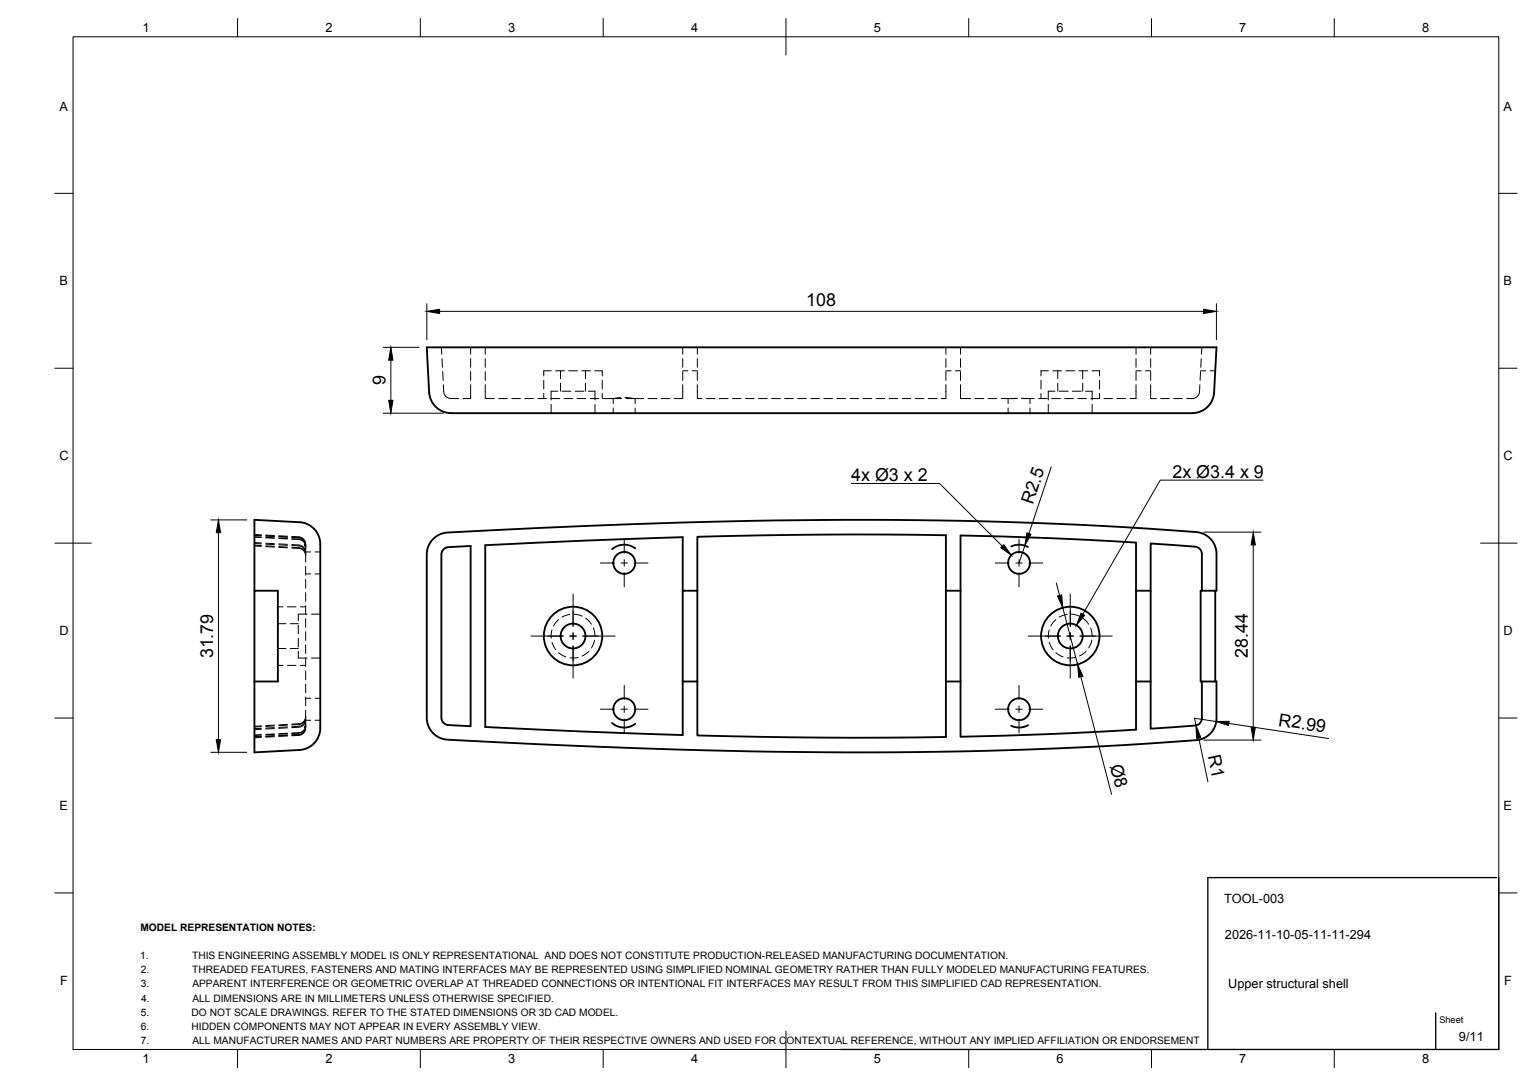
ISO-10303-21;
HEADER;
/* Generated by software containing ST-Developer
 * from STEP Tools, Inc. (www.steptools.com) 
 */

FILE_DESCRIPTION(
/* description */ (''),
/* implementation_level */ '2;1');

FILE_NAME(
/* name */ 'Upper structural shell.step',
/* time_stamp */ '2026-11-10T05:20:16-08:00',
/* author */ (''),
/* organization */ (''),
/* preprocessor_version */ 'ST-DEVELOPER v20.2',
/* originating_system */ 'Autodesk Translation Framework v15.17.0.0',
/* authorisation */ '');

FILE_SCHEMA (('AUTOMOTIVE_DESIGN { 1 0 10303 214 3 1 1 }'));
ENDSEC;

DATA;
#10=MECHANICAL_DESIGN_GEOMETRIC_PRESENTATION_REPRESENTATION('',(#116),#24809);
#76=SPHERICAL_SURFACE('',#10334,0.1);
#77=SPHERICAL_SURFACE('',#10337,0.0999999999999998);
#78=SPHERICAL_SURFACE('',#10341,0.0999999999999993);
#79=SPHERICAL_SURFACE('',#10345,0.1);
#80=SPHERICAL_SURFACE('',#10350,0.3);
#81=SPHERICAL_SURFACE('',#10354,0.3);
#82=SPHERICAL_SURFACE('',#10358,0.299999999999999);
#83=SPHERICAL_SURFACE('',#10363,0.3);
#96=SHAPE_REPRESENTATION_RELATIONSHIP('SRR','None',#24860,#106);
#106=ADVANCED_BREP_SHAPE_REPRESENTATION('',(#126),#24803);
#116=STYLED_ITEM('',(#24922),#126);
#126=MANIFOLD_SOLID_BREP('Body1',#9893);
#147=FACE_BOUND('',#2104,.T.);
#148=FACE_BOUND('',#2105,.T.);
#149=FACE_BOUND('',#2106,.T.);
#150=FACE_BOUND('',#2113,.T.);
#151=FACE_BOUND('',#2116,.T.);
#152=FACE_BOUND('',#2127,.T.);
#153=FACE_BOUND('',#2129,.T.);
#154=FACE_BOUND('',#2141,.T.);
#155=FACE_BOUND('',#2162,.T.);
#156=FACE_BOUND('',#2163,.T.);
#157=FACE_BOUND('',#2164,.T.);
#158=FACE_BOUND('',#2199,.T.);
#159=FACE_BOUND('',#2200,.T.);
#160=FACE_BOUND('',#2201,.T.);
#161=FACE_BOUND('',#2202,.T.);
#162=FACE_BOUND('',#2203,.T.);
#163=FACE_BOUND('',#2204,.T.);
#205=B_SPLINE_SURFACE_WITH_KNOTS('',3,3,((#15043,#15044,#15045,#15046),
(#15047,#15048,#15049,#15050),(#15051,#15052,#15053,#15054),(#15055,#15056,
#15057,#15058),(#15059,#15060,#15061,#15062)),.UNSPECIFIED.,.F.,.F.,.F.,
(4,1,4),(4,4),(0.,0.571428571428571,1.),(1.0454440030657,3.44967454744645),
 .UNSPECIFIED.);
#206=B_SPLINE_SURFACE_WITH_KNOTS('',3,3,((#15135,#15136,#15137,#15138),
(#15139,#15140,#15141,#15142),(#15143,#15144,#15145,#15146),(#15147,#15148,
#15149,#15150),(#15151,#15152,#15153,#15154)),.UNSPECIFIED.,.F.,.F.,.F.,
(4,1,4),(4,4),(0.,0.571428571428571,1.),(7.24519303641511,9.95046872158573),
 .UNSPECIFIED.);
#207=B_SPLINE_SURFACE_WITH_KNOTS('',3,3,((#16016,#16017,#16018,#16019),
(#16020,#16021,#16022,#16023),(#16024,#16025,#16026,#16027),(#16028,#16029,
#16030,#16031)),.UNSPECIFIED.,.F.,.F.,.F.,(4,4),(4,4),(0.0705535719740953,
0.323522444336189),(0.0117434863834119,0.684857763552191),.UNSPECIFIED.);
#208=B_SPLINE_SURFACE_WITH_KNOTS('',3,3,((#16036,#16037,#16038,#16039),
(#16040,#16041,#16042,#16043),(#16044,#16045,#16046,#16047),(#16048,#16049,
#16050,#16051)),.UNSPECIFIED.,.F.,.F.,.F.,(4,4),(4,4),(0.0262419052680539,
0.0545428296147404),(0.0121538053864343,0.684980602226481),
 .UNSPECIFIED.);
#209=B_SPLINE_SURFACE_WITH_KNOTS('',3,3,((#16061,#16062,#16063,#16064),
(#16065,#16066,#16067,#16068),(#16069,#16070,#16071,#16072),(#16073,#16074,
#16075,#16076),(#16077,#16078,#16079,#16080)),.UNSPECIFIED.,.F.,.F.,.F.,
(4,1,4),(4,4),(0.,0.571428571428571,1.),(0.752061768057538,3.45733745322815),
 .UNSPECIFIED.);
#210=B_SPLINE_SURFACE_WITH_KNOTS('',3,3,((#16081,#16082,#16083,#16084),
(#16085,#16086,#16087,#16088),(#16089,#16090,#16091,#16092),(#16093,#16094,
#16095,#16096),(#16097,#16098,#16099,#16100)),.UNSPECIFIED.,.F.,.F.,.F.,
(4,1,4),(4,4),(0.,0.571428571428571,1.),(0.283259008618247,0.557056952888827),
 .UNSPECIFIED.);
#211=B_SPLINE_SURFACE_WITH_KNOTS('',3,3,((#16114,#16115,#16116,#16117),
(#16118,#16119,#16120,#16121),(#16122,#16123,#16124,#16125),(#16126,#16127,
#16128,#16129)),.UNSPECIFIED.,.F.,.F.,.F.,(4,4),(4,4),(0.67647755566375,
0.929446428026011),(0.0117434863436937,0.684857763580381),.UNSPECIFIED.);
#212=B_SPLINE_SURFACE_WITH_KNOTS('',3,3,((#16130,#16131,#16132,#16133),
(#16134,#16135,#16136,#16137),(#16138,#16139,#16140,#16141),(#16142,#16143,
#16144,#16145)),.UNSPECIFIED.,.F.,.F.,.F.,(4,4),(4,4),(0.945457170385156,
0.973758094731946),(0.0121538053598088,0.684980602226481),.UNSPECIFIED.);
#213=B_SPLINE_SURFACE_WITH_KNOTS('',3,3,((#16229,#16230,#16231,#16232),
(#16233,#16234,#16235,#16236),(#16237,#16238,#16239,#16240),(#16241,#16242,
#16243,#16244)),.UNSPECIFIED.,.F.,.F.,.F.,(4,4),(4,4),(0.341142793678372,
0.658675488550287),(0.0116221239297273,0.684255166525269),.UNSPECIFIED.);
#214=B_SPLINE_SURFACE_WITH_KNOTS('',3,3,((#16249,#16250,#16251,#16252),
(#16253,#16254,#16255,#16256),(#16257,#16258,#16259,#16260),(#16261,#16262,
#16263,#16264),(#16265,#16266,#16267,#16268)),.UNSPECIFIED.,.F.,.F.,.F.,
(4,1,4),(4,4),(0.,0.571428571428571,1.),(3.65450559744172,7.0548588409572),
 .UNSPECIFIED.);
#215=B_SPLINE_SURFACE_WITH_KNOTS('',3,3,((#16278,#16279,#16280,#16281),
(#16282,#16283,#16284,#16285),(#16286,#16287,#16288,#16289),(#16290,#16291,
#16292,#16293),(#16294,#16295,#16296,#16297)),.UNSPECIFIED.,.F.,.F.,.F.,
(4,1,4),(4,4),(0.,0.571428571428571,1.),(3.64767164868607,7.04802489220155),
 .UNSPECIFIED.);
#216=B_SPLINE_SURFACE_WITH_KNOTS('',3,3,((#16302,#16303,#16304,#16305),
(#16306,#16307,#16308,#16309),(#16310,#16311,#16312,#16313),(#16314,#16315,
#16316,#16317)),.UNSPECIFIED.,.F.,.F.,.F.,(4,4),(4,4),(0.341324511449716,
0.658857206321627),(0.0116221214776208,0.684255166525269),.UNSPECIFIED.);
#217=B_SPLINE_SURFACE_WITH_KNOTS('',3,3,((#16362,#16363,#16364,#16365),
(#16366,#16367,#16368,#16369),(#16370,#16371,#16372,#16373),(#16374,#16375,
#16376,#16377)),.UNSPECIFIED.,.F.,.F.,.F.,(4,4),(4,4),(0.676316266718331,
0.901708040522105),(0.0117102006467275,0.68495201331719),.UNSPECIFIED.);
#218=B_SPLINE_SURFACE_WITH_KNOTS('',3,3,((#16382,#16383,#16384,#16385),
(#16386,#16387,#16388,#16389),(#16390,#16391,#16392,#16393),(#16394,#16395,
#16396,#16397),(#16398,#16399,#16400,#16401)),.UNSPECIFIED.,.F.,.F.,.F.,
(4,1,4),(4,4),(0.,0.571428571428571,1.),(7.25285594219682,9.65708648657758),
 .UNSPECIFIED.);
#219=B_SPLINE_SURFACE_WITH_KNOTS('',3,3,((#16411,#16412,#16413,#16414),
(#16415,#16416,#16417,#16418),(#16419,#16420,#16421,#16422),(#16423,#16424,
#16425,#16426)),.UNSPECIFIED.,.F.,.F.,.F.,(4,4),(4,4),(0.0982919594778951,
0.323683733281714),(0.0117102006467272,0.68495201331719),.UNSPECIFIED.);
#220=B_SPLINE_SURFACE_WITH_KNOTS('',3,3,((#16501,#16502,#16503,#16504),
(#16505,#16506,#16507,#16508),(#16509,#16510,#16511,#16512),(#16513,#16514,
#16515,#16516)),.UNSPECIFIED.,.F.,.F.,.F.,(4,4),(4,4),(0.917922863855343,
0.974411608827007),(0.0122403473423911,0.685344304754238),.UNSPECIFIED.);
#221=B_SPLINE_SURFACE_WITH_KNOTS('',3,3,((#16526,#16527,#16528,#16529),
(#16530,#16531,#16532,#16533),(#16534,#16535,#16536,#16537),(#16538,#16539,
#16540,#16541),(#16542,#16543,#16544,#16545)),.UNSPECIFIED.,.F.,.F.,.F.,
(4,1,4),(4,4),(0.,0.571428571428571,1.),(9.85085636625011,10.4271318523291),
 .UNSPECIFIED.);
#222=B_SPLINE_SURFACE_WITH_KNOTS('',3,3,((#16559,#16560,#16561,#16562),
(#16563,#16564,#16565,#16566),(#16567,#16568,#16569,#16570),(#16571,#16572,
#16573,#16574)),.UNSPECIFIED.,.F.,.F.,.F.,(4,4),(4,4),(0.025588391172993,
0.0820771361446569),(0.0122403473423911,0.685344304754238),
 .UNSPECIFIED.);
#223=B_SPLINE_SURFACE_WITH_KNOTS('',3,3,((#16584,#16585,#16586,#16587),
(#16588,#16589,#16590,#16591),(#16592,#16593,#16594,#16595),(#16596,#16597,
#16598,#16599),(#16600,#16601,#16602,#16603)),.UNSPECIFIED.,.F.,.F.,.F.,
(4,1,4),(4,4),(0.,0.571428571428571,1.),(0.27539863731415,0.851674123393175),
 .UNSPECIFIED.);
#224=B_SPLINE_SURFACE_WITH_KNOTS('',3,3,((#16617,#16618,#16619,#16620),
(#16621,#16622,#16623,#16624),(#16625,#16626,#16627,#16628),(#16629,#16630,
#16631,#16632),(#16633,#16634,#16635,#16636)),.UNSPECIFIED.,.F.,.F.,.F.,
(4,1,4),(4,4),(0.,0.571428571428571,1.),(0.00944995813270487,0.618489359031386),
 .UNSPECIFIED.);
#225=B_SPLINE_SURFACE_WITH_KNOTS('',3,3,((#16643,#16644,#16645,#16646),
(#16647,#16648,#16649,#16650),(#16651,#16652,#16653,#16654),(#16655,#16656,
#16657,#16658),(#16659,#16660,#16661,#16662)),.UNSPECIFIED.,.F.,.F.,.F.,
(4,1,4),(4,4),(0.,0.571428571428571,1.),(0.00908570715245136,0.618164468641375),
 .UNSPECIFIED.);
#226=B_SPLINE_SURFACE_WITH_KNOTS('',3,3,((#16667,#16668,#16669,#16670),
(#16671,#16672,#16673,#16674),(#16675,#16676,#16677,#16678),(#16679,#16680,
#16681,#16682),(#16683,#16684,#16685,#16686)),.UNSPECIFIED.,.F.,.F.,.F.,
(4,1,4),(4,4),(0.,0.571428571428571,1.),(0.0091183540525243,0.618164468641375),
 .UNSPECIFIED.);
#227=B_SPLINE_SURFACE_WITH_KNOTS('',3,3,((#16691,#16692,#16693,#16694),
(#16695,#16696,#16697,#16698),(#16699,#16700,#16701,#16702),(#16703,#16704,
#16705,#16706),(#16707,#16708,#16709,#16710)),.UNSPECIFIED.,.F.,.F.,.F.,
(4,1,4),(4,4),(0.,0.571428571428571,1.),(10.1454735367545,10.419271481025),
 .UNSPECIFIED.);
#228=B_SPLINE_SURFACE_WITH_KNOTS('',3,3,((#16711,#16712,#16713,#16714),
(#16715,#16716,#16717,#16718),(#16719,#16720,#16721,#16722),(#16723,#16724,
#16725,#16726),(#16727,#16728,#16729,#16730)),.UNSPECIFIED.,.F.,.F.,.F.,
(4,1,4),(4,4),(0.,0.571428571428571,1.),(0.0094045468285345,0.618489359031386),
 .UNSPECIFIED.);
#229=B_SPLINE_SURFACE_WITH_KNOTS('',3,3,((#16756,#16757,#16758,#16759),
(#16760,#16761,#16762,#16763),(#16764,#16765,#16766,#16767),(#16768,#16769,
#16770,#16771),(#16772,#16773,#16774,#16775)),.UNSPECIFIED.,.F.,.F.,.F.,
(4,1,4),(4,4),(0.,0.571428571428571,1.),(-0.00535061636073277,0.618489359031386),
 .UNSPECIFIED.);
#230=B_SPLINE_SURFACE_WITH_KNOTS('',3,3,((#16794,#16795,#16796,#16797,#16798),
(#16799,#16800,#16801,#16802,#16803),(#16804,#16805,#16806,#16807,#16808),
(#16809,#16810,#16811,#16812,#16813),(#16814,#16815,#16816,#16817,#16818)),
 .UNSPECIFIED.,.F.,.F.,.F.,(4,1,4),(4,1,4),(0.,0.571428571428571,1.),(0.283259008618247,
4.63063308449434,10.4271318523291),.UNSPECIFIED.);
#231=B_SPLINE_SURFACE_WITH_KNOTS('',3,3,((#16829,#16830,#16831,#16832),
(#16833,#16834,#16835,#16836),(#16837,#16838,#16839,#16840),(#16841,#16842,
#16843,#16844),(#16845,#16846,#16847,#16848)),.UNSPECIFIED.,.F.,.F.,.F.,
(4,1,4),(4,4),(0.,0.571428571428571,1.),(-0.00578978989683084,0.618164468641375),
 .UNSPECIFIED.);
#232=B_SPLINE_SURFACE_WITH_KNOTS('',3,3,((#16857,#16858,#16859,#16860),
(#16861,#16862,#16863,#16864),(#16865,#16866,#16867,#16868),(#16869,#16870,
#16871,#16872),(#16873,#16874,#16875,#16876)),.UNSPECIFIED.,.F.,.F.,.F.,
(4,1,4),(4,4),(0.,0.571428571428571,1.),(-0.00569189159989896,0.618164468641375),
 .UNSPECIFIED.);
#233=B_SPLINE_SURFACE_WITH_KNOTS('',3,3,((#16885,#16886,#16887,#16888,#16889),
(#16890,#16891,#16892,#16893,#16894),(#16895,#16896,#16897,#16898,#16899),
(#16900,#16901,#16902,#16903,#16904),(#16905,#16906,#16907,#16908,#16909)),
 .UNSPECIFIED.,.F.,.F.,.F.,(4,1,4),(4,1,4),(0.,0.571428571428571,1.),(0.27539863731415,
4.62277271319024,10.419271481025),.UNSPECIFIED.);
#234=B_SPLINE_SURFACE_WITH_KNOTS('',3,3,((#16920,#16921,#16922,#16923),
(#16924,#16925,#16926,#16927),(#16928,#16929,#16930,#16931),(#16932,#16933,
#16934,#16935),(#16936,#16937,#16938,#16939)),.UNSPECIFIED.,.F.,.F.,.F.,
(4,1,4),(4,4),(0.,0.571428571428571,1.),(-0.0054868135546625,0.618489359031386),
 .UNSPECIFIED.);
#235=B_SPLINE_SURFACE_WITH_KNOTS('',3,3,((#16948,#16949,#16950,#16951),
(#16952,#16953,#16954,#16955),(#16956,#16957,#16958,#16959),(#16960,#16961,
#16962,#16963)),.UNSPECIFIED.,.F.,.F.,.F.,(4,4),(4,4),(0.026239262514127,
0.974414173651419),(0.,0.685344304754238),.UNSPECIFIED.);
#236=B_SPLINE_SURFACE_WITH_KNOTS('',3,3,((#16966,#16967,#16968,#16969),
(#16970,#16971,#16972,#16973),(#16974,#16975,#16976,#16977),(#16978,#16979,
#16980,#16981)),.UNSPECIFIED.,.F.,.F.,.F.,(4,4),(4,4),(0.0255858263485814,
0.973760737485873),(0.,0.685344304754238),.UNSPECIFIED.);
#617=B_SPLINE_CURVE_WITH_KNOTS('',3,(#14942,#14943,#14944,#14945,#14946,
#14947,#14948,#14949,#14950,#14951,#14952,#14953,#14954,#14955,#14956,#14957,
#14958,#14959,#14960,#14961,#14962,#14963,#14964,#14965),.UNSPECIFIED.,
 .F.,.F.,(4,2,2,2,2,2,2,2,2,2,2,4),(-0.337265338267783,-0.250544943628509,
-0.208272806508042,-0.186542211788094,-0.176382978682897,-0.170925844043069,
-0.16639450677335,-0.161077381235501,-0.15182241135393,-0.115009181549223,
-0.030206004227969,0.),.UNSPECIFIED.);
#618=B_SPLINE_CURVE_WITH_KNOTS('',3,(#14970,#14971,#14972,#14973,#14974,
#14975,#14976,#14977,#14978,#14979,#14980,#14981,#14982,#14983,#14984,#14985,
#14986,#14987,#14988,#14989),.UNSPECIFIED.,.F.,.F.,(4,2,2,2,2,2,2,2,2,4),
(-0.240982594686416,-0.16829976149504,-0.141836598208813,-0.129116059226128,
-0.121962912034391,-0.115857591426886,-0.108506552485159,-0.0948769875819265,
-0.0364654790774683,0.),.UNSPECIFIED.);
#619=B_SPLINE_CURVE_WITH_KNOTS('',3,(#14994,#14995,#14996,#14997,#14998,
#14999,#15000,#15001,#15002,#15003,#15004,#15005,#15006,#15007,#15008,#15009,
#15010,#15011,#15012,#15013),.UNSPECIFIED.,.F.,.F.,(4,2,2,2,2,2,2,2,2,4),
(-0.240981214998207,-0.168303541671295,-0.141841407502325,-0.129121097580905,
-0.121968013294536,-0.115862708924237,-0.108511643765797,-0.0948818976588229,
-0.0364681276985956,0.),.UNSPECIFIED.);
#620=B_SPLINE_CURVE_WITH_KNOTS('',3,(#15018,#15019,#15020,#15021,#15022,
#15023,#15024,#15025,#15026,#15027,#15028,#15029,#15030,#15031,#15032,#15033,
#15034,#15035,#15036,#15037,#15038,#15039,#15040,#15041),.UNSPECIFIED.,
 .F.,.F.,(4,2,2,2,2,2,2,2,2,2,2,4),(-0.337269388373684,-0.250545316912909,
-0.208282401844766,-0.186554569827561,-0.176396213396297,-0.17093921790305,
-0.16640782243471,-0.161090427650893,-0.151834477986603,-0.115010808423941,
-0.0302102096065556,0.),.UNSPECIFIED.);
#621=B_SPLINE_CURVE_WITH_KNOTS('',3,(#15064,#15065,#15066,#15067),
 .UNSPECIFIED.,.F.,.F.,(4,4),(1.0454440030657,2.52465537163019),
 .UNSPECIFIED.);
#622=B_SPLINE_CURVE_WITH_KNOTS('',3,(#15069,#15070,#15071,#15072,#15073,
#15074,#15075,#15076,#15077,#15078,#15079,#15080,#15081,#15082,#15083,#15084,
#15085,#15086,#15087,#15088,#15089,#15090,#15091,#15092,#15093,#15094,#15095,
#15096),.UNSPECIFIED.,.F.,.F.,(4,3,3,3,3,3,3,3,3,4),(-0.152193408756968,
-0.128427023368412,-0.115107736263918,-0.0911810900745799,-0.0780377802127556,
-0.0652031397886901,-0.0414031558437525,-0.0389949527774582,-0.0152076153333754,
0.),.UNSPECIFIED.);
#623=B_SPLINE_CURVE_WITH_KNOTS('',3,(#15098,#15099,#15100,#15101),
 .UNSPECIFIED.,.F.,.F.,(4,4),(-3.44967454744645,-1.05170160817356),
 .UNSPECIFIED.);
#624=B_SPLINE_CURVE_WITH_KNOTS('',3,(#15103,#15104,#15105,#15106,#15107,
#15108,#15109,#15110,#15111,#15112,#15113,#15114,#15115,#15116,#15117,#15118,
#15119,#15120,#15121,#15122,#15123,#15124,#15125,#15126,#15127,#15128,#15129,
#15130),.UNSPECIFIED.,.F.,.F.,(4,3,3,3,3,3,3,3,3,4),(-0.152278960443096,
-0.128503570101575,-0.115218572146868,-0.09145408274965,-0.0870214650669139,
-0.0781562978024333,-0.0542566895399357,-0.03908030849237,-0.0153296112319379,
0.),.UNSPECIFIED.);
#625=B_SPLINE_CURVE_WITH_KNOTS('',3,(#15131,#15132,#15133,#15134),
 .UNSPECIFIED.,.F.,.F.,(4,4),(2.75501813708031,3.4476340663212),
 .UNSPECIFIED.);
#626=B_SPLINE_CURVE_WITH_KNOTS('',3,(#15156,#15157,#15158,#15159),
 .UNSPECIFIED.,.F.,.F.,(4,4),(7.24810383506675,7.89761558728778),
 .UNSPECIFIED.);
#627=B_SPLINE_CURVE_WITH_KNOTS('',3,(#15161,#15162,#15163,#15164,#15165,
#15166,#15167,#15168,#15169,#15170,#15171,#15172,#15173,#15174,#15175,#15176,
#15177,#15178,#15179,#15180,#15181,#15182,#15183,#15184,#15185,#15186,#15187,
#15188),.UNSPECIFIED.,.F.,.F.,(4,3,3,3,3,3,3,3,3,4),(-0.152278869104567,
-0.128548794904564,-0.115192257893812,-0.0912773536606376,-0.0781090575823055,
-0.0652724057916263,-0.0414819581560496,-0.0390493575290778,-0.015259721743698,
0.),.UNSPECIFIED.);
#628=B_SPLINE_CURVE_WITH_KNOTS('',3,(#15190,#15191,#15192,#15193),
 .UNSPECIFIED.,.F.,.F.,(4,4),(-9.94532343034734,-7.24519303641511),
 .UNSPECIFIED.);
#629=B_SPLINE_CURVE_WITH_KNOTS('',3,(#15195,#15196,#15197,#15198,#15199,
#15200,#15201,#15202,#15203,#15204,#15205,#15206,#15207,#15208,#15209,#15210,
#15211,#15212,#15213,#15214,#15215,#15216,#15217,#15218,#15219,#15220,#15221,
#15222),.UNSPECIFIED.,.F.,.F.,(4,3,3,3,3,3,3,3,3,4),(-0.152181623618259,
-0.128410404494075,-0.115248188224843,-0.0914746846046984,-0.0869904866333268,
-0.0783028696190655,-0.0543945376065823,-0.0391651209697638,-0.0153884182770307,
0.),.UNSPECIFIED.);
#630=B_SPLINE_CURVE_WITH_KNOTS('',3,(#15223,#15224,#15225,#15226),
 .UNSPECIFIED.,.F.,.F.,(4,4),(8.21380824320284,9.95046871680089),
 .UNSPECIFIED.);
#631=B_SPLINE_CURVE_WITH_KNOTS('',3,(#15229,#15230,#15231,#15232),
 .UNSPECIFIED.,.F.,.F.,(4,4),(2.80491490332713,3.45442665446657),
 .UNSPECIFIED.);
#632=B_SPLINE_CURVE_WITH_KNOTS('',3,(#15236,#15237,#15238,#15239),
 .UNSPECIFIED.,.F.,.F.,(4,4),(0.752061768057538,2.48872224644044),
 .UNSPECIFIED.);
#633=B_SPLINE_CURVE_WITH_KNOTS('',3,(#15387,#15388,#15389,#15390,#15391,
#15392),.UNSPECIFIED.,.F.,.F.,(4,2,4),(-0.606700505977711,-0.303383635264422,
-0.000339350725729326),.UNSPECIFIED.);
#634=B_SPLINE_CURVE_WITH_KNOTS('',3,(#15393,#15394,#15395,#15396,#15397,
#15398,#15399,#15400,#15401,#15402,#15403,#15404,#15405,#15406,#15407,#15408,
#15409,#15410,#15411,#15412,#15413,#15414,#15415,#15416,#15417,#15418,#15419,
#15420),.UNSPECIFIED.,.F.,.F.,(4,3,3,3,3,3,3,3,3,4),(-0.152173579228948,
-0.128423230539522,-0.115115104157663,-0.0911927259648815,-0.0780672068328041,
-0.0652082609452843,-0.0414117413801899,-0.0390174000215468,-0.0152300060615686,
0.),.UNSPECIFIED.);
#635=B_SPLINE_CURVE_WITH_KNOTS('',3,(#15421,#15422,#15423,#15424,#15425,
#15426),.UNSPECIFIED.,.F.,.F.,(4,2,4),(-0.606471894652381,-0.303383500305553,
-0.00011071898471493),.UNSPECIFIED.);
#636=B_SPLINE_CURVE_WITH_KNOTS('',3,(#15430,#15431,#15432,#15433,#15434,
#15435),.UNSPECIFIED.,.F.,.F.,(4,2,4),(-0.606240625011114,-0.303433113375332,
-0.00010938105916114),.UNSPECIFIED.);
#637=B_SPLINE_CURVE_WITH_KNOTS('',3,(#15437,#15438,#15439,#15440,#15441,
#15442,#15443,#15444,#15445,#15446,#15447,#15448,#15449,#15450,#15451,#15452,
#15453,#15454,#15455,#15456,#15457,#15458,#15459,#15460,#15461,#15462,#15463,
#15464),.UNSPECIFIED.,.F.,.F.,(4,3,3,3,3,3,3,3,3,4),(-0.152281454644235,
-0.128508102092242,-0.115234945630277,-0.0914677943501604,-0.0870276017853555,
-0.0781846052914712,-0.0542821334115454,-0.0390966859411886,-0.0153419673568312,
0.),.UNSPECIFIED.);
#638=B_SPLINE_CURVE_WITH_KNOTS('',3,(#15466,#15467,#15468,#15469,#15470,
#15471),.UNSPECIFIED.,.F.,.F.,(4,2,4),(-0.606758573154242,-0.303433157101101,
-0.000627306481538803),.UNSPECIFIED.);
#639=B_SPLINE_CURVE_WITH_KNOTS('',3,(#15477,#15478,#15479,#15480,#15481,
#15482),.UNSPECIFIED.,.F.,.F.,(4,2,4),(-0.60617382748,-0.303436117212405,
-7.2700296824213E-5),.UNSPECIFIED.);
#640=B_SPLINE_CURVE_WITH_KNOTS('',3,(#15484,#15485,#15486,#15487,#15488,
#15489,#15490,#15491,#15492,#15493,#15494,#15495,#15496,#15497,#15498,#15499,
#15500,#15501,#15502,#15503,#15504,#15505,#15506,#15507,#15508,#15509,#15510,
#15511),.UNSPECIFIED.,.F.,.F.,(4,3,3,3,3,3,3,3,3,4),(-0.152282154327755,
-0.128558036203745,-0.115201429639692,-0.0912891813973639,-0.0781219052297615,
-0.065279687589213,-0.0414913146723999,-0.0390591331507366,-0.0152683745546824,
0.),.UNSPECIFIED.);
#641=B_SPLINE_CURVE_WITH_KNOTS('',3,(#15515,#15516,#15517,#15518,#15519,
#15520,#15521,#15522,#15523,#15524,#15525,#15526,#15527,#15528,#15529,#15530,
#15531,#15532,#15533,#15534,#15535,#15536,#15537,#15538,#15539,#15540,#15541,
#15542),.UNSPECIFIED.,.F.,.F.,(4,3,3,3,3,3,3,3,3,4),(-0.152283066055976,
-0.128508717930245,-0.115216472798554,-0.091451700383826,-0.087022506454752,
-0.0781485278686168,-0.0542483994686567,-0.0390758108455304,-0.0153274175274101,
0.),.UNSPECIFIED.);
#642=B_SPLINE_CURVE_WITH_KNOTS('',3,(#15544,#15545,#15546,#15547,#15548,
#15549),.UNSPECIFIED.,.F.,.F.,(4,2,4),(-0.606800264911061,-0.303436147592132,
-0.000699137727853738),.UNSPECIFIED.);
#643=B_SPLINE_CURVE_WITH_KNOTS('',3,(#15554,#15555,#15556,#15557,#15558,
#15559),.UNSPECIFIED.,.F.,.F.,(4,2,4),(-0.606915279655722,-0.30363236403835,
-0.000516487074480598),.UNSPECIFIED.);
#644=B_SPLINE_CURVE_WITH_KNOTS('',3,(#15563,#15564,#15565,#15566,#15567,
#15568,#15569,#15570,#15571,#15572,#15573,#15574,#15575,#15576,#15577,#15578,
#15579,#15580,#15581,#15582,#15583,#15584,#15585,#15586,#15587,#15588,#15589,
#15590),.UNSPECIFIED.,.F.,.F.,(4,3,3,3,3,3,3,3,3,4),(-0.152205325335401,
-0.128433618138404,-0.115304790388008,-0.091527299141506,-0.0870178586418932,
-0.0783866443643876,-0.0544751548276533,-0.0392137310602028,-0.0154203878854647,
0.),.UNSPECIFIED.);
#645=B_SPLINE_CURVE_WITH_KNOTS('',3,(#15592,#15593,#15594,#15595,#15596,
#15597),.UNSPECIFIED.,.F.,.F.,(4,2,4),(-0.606752424187958,-0.303632696349781,
-0.000353591088346872),.UNSPECIFIED.);
#646=B_SPLINE_CURVE_WITH_KNOTS('',3,(#15603,#15604,#15605,#15606),
 .UNSPECIFIED.,.F.,.F.,(4,4),(0.0116023361771303,0.618489359031386),
 .UNSPECIFIED.);
#647=B_SPLINE_CURVE_WITH_KNOTS('',3,(#15610,#15611,#15612,#15613),
 .UNSPECIFIED.,.F.,.F.,(4,4),(-0.618489359031386,-0.01160233617713),
 .UNSPECIFIED.);
#648=B_SPLINE_CURVE_WITH_KNOTS('',3,(#15616,#15617,#15618,#15619),
 .UNSPECIFIED.,.F.,.F.,(4,4),(7.01593971618694,9.71770560667459),
 .UNSPECIFIED.);
#649=B_SPLINE_CURVE_WITH_KNOTS('',3,(#15620,#15621,#15622,#15623),
 .UNSPECIFIED.,.F.,.F.,(4,4),(0.505945342046796,3.20718651982575),
 .UNSPECIFIED.);
#650=B_SPLINE_CURVE_WITH_KNOTS('',3,(#15626,#15627,#15628,#15629,#15630,
#15631,#15632),.UNSPECIFIED.,.F.,.F.,(4,3,4),(3.40717417387402,5.11170895874517,
6.80746068626633),.UNSPECIFIED.);
#651=B_SPLINE_CURVE_WITH_KNOTS('',3,(#15635,#15636,#15637,#15638),
 .UNSPECIFIED.,.F.,.F.,(4,4),(7.00766573366377,9.41198845520559),
 .UNSPECIFIED.);
#652=B_SPLINE_CURVE_WITH_KNOTS('',3,(#15642,#15643,#15644,#15645),
 .UNSPECIFIED.,.F.,.F.,(4,4),(9.61248784142317,10.2217363065808),
 .UNSPECIFIED.);
#653=B_SPLINE_CURVE_WITH_KNOTS('',3,(#15646,#15647,#15648,#15649,#15650,
#15651,#15652,#15653,#15654,#15655,#15656,#15657,#15658,#15659,#15660,#15661,
#15662,#15663,#15664,#15665,#15666,#15667,#15668,#15669,#15670,#15671,#15672,
#15673),.UNSPECIFIED.,.F.,.F.,(4,3,3,3,3,3,3,3,3,4),(0.,0.0238103109064959,
0.0390781362249314,0.0628635086275546,0.0641230352384255,0.0780643700703951,
0.101962174814111,0.113803522271848,0.137549611554782,0.149564734365165),
 .UNSPECIFIED.);
#654=B_SPLINE_CURVE_WITH_KNOTS('',3,(#15677,#15678,#15679,#15680,#15681,
#15682,#15683,#15684,#15685,#15686,#15687,#15688,#15689,#15690,#15691,#15692,
#15693,#15694,#15695,#15696,#15697,#15698,#15699,#15700,#15701,#15702,#15703,
#15704,#15705,#15706,#15707),.UNSPECIFIED.,.F.,.F.,(4,3,3,3,3,3,3,3,3,3,
4),(0.,0.0535521515156599,0.107729685495911,0.117233338918226,0.171447998942947,
0.1923696899792,0.234191611538245,0.288659693466396,0.341410301570312,0.395549383747909,
0.448696573746633),.UNSPECIFIED.);
#655=B_SPLINE_CURVE_WITH_KNOTS('',3,(#15709,#15710,#15711,#15712),
 .UNSPECIFIED.,.F.,.F.,(4,4),(0.0255858263485814,0.973760737485873),
 .UNSPECIFIED.);
#656=B_SPLINE_CURVE_WITH_KNOTS('',3,(#15714,#15715,#15716,#15717,#15718,
#15719,#15720,#15721,#15722,#15723,#15724,#15725,#15726,#15727,#15728,#15729,
#15730,#15731,#15732,#15733,#15734,#15735,#15736,#15737,#15738,#15739,#15740,
#15741,#15742,#15743,#15744),.UNSPECIFIED.,.F.,.F.,(4,3,3,3,3,3,3,3,3,3,
4),(0.,0.0535144560117858,0.107726856902975,0.117300577410231,0.171517675930231,
0.195438847090422,0.234297456941738,0.289665153342662,0.345032849743585,
0.40043206955427,0.455831289364955),.UNSPECIFIED.);
#657=B_SPLINE_CURVE_WITH_KNOTS('',3,(#15748,#15749,#15750,#15751,#15752,
#15753,#15754,#15755,#15756,#15757,#15758,#15759,#15760,#15761,#15762,#15763,
#15764,#15765,#15766,#15767,#15768,#15769,#15770,#15771,#15772,#15773,#15774,
#15775,#15776,#15777,#15778),.UNSPECIFIED.,.F.,.F.,(4,3,3,3,3,3,3,3,3,3,
4),(0.,0.053505543180391,0.107714168832353,0.117253997025819,0.171473395203321,
0.195418854185489,0.234223199196375,0.289607016015183,0.344990832833991,
0.400409777473312,0.455828722112633),.UNSPECIFIED.);
#658=B_SPLINE_CURVE_WITH_KNOTS('',3,(#15780,#15781,#15782,#15783),
 .UNSPECIFIED.,.F.,.F.,(4,4),(0.0262392625141271,0.974414173651419),
 .UNSPECIFIED.);
#659=B_SPLINE_CURVE_WITH_KNOTS('',3,(#15785,#15786,#15787,#15788,#15789,
#15790,#15791,#15792,#15793,#15794,#15795,#15796,#15797,#15798,#15799,#15800,
#15801,#15802,#15803,#15804,#15805,#15806,#15807,#15808,#15809,#15810,#15811,
#15812,#15813,#15814,#15815),.UNSPECIFIED.,.F.,.F.,(4,3,3,3,3,3,3,3,3,3,
4),(0.,0.0535648734523888,0.107747221190676,0.117299947751206,0.171510987106922,
0.192397607227928,0.234296687348373,0.288768001369001,0.341469499352622,
0.395597672314973,0.448700135162036),.UNSPECIFIED.);
#660=B_SPLINE_CURVE_WITH_KNOTS('',3,(#15818,#15819,#15820,#15821,#15822,
#15823,#15824,#15825,#15826,#15827,#15828,#15829,#15830,#15831,#15832,#15833,
#15834,#15835,#15836,#15837,#15838,#15839,#15840,#15841,#15842),
 .UNSPECIFIED.,.F.,.F.,(4,3,3,3,3,3,3,3,4),(0.,0.0238141989470671,0.0391004231578824,
0.0641320992313133,0.0780996136084711,0.101998806889826,0.113823260594808,
0.137564745199532,0.149565921982294),.UNSPECIFIED.);
#661=B_SPLINE_CURVE_WITH_KNOTS('',3,(#15844,#15845,#15846,#15847),
 .UNSPECIFIED.,.F.,.F.,(4,4),(2.76692059912875E-5,0.609394470571143),
 .UNSPECIFIED.);
#662=B_SPLINE_CURVE_WITH_KNOTS('',3,(#15850,#15851,#15852,#15853),
 .UNSPECIFIED.,.F.,.F.,(4,4),(0.809932799154201,3.21472245120952),
 .UNSPECIFIED.);
#663=B_SPLINE_CURVE_WITH_KNOTS('',3,(#15856,#15857,#15858,#15859,#15860,
#15861,#15862),.UNSPECIFIED.,.F.,.F.,(4,3,4),(3.41496637450242,5.11093193409745,
6.81591321610411),.UNSPECIFIED.);
#664=B_SPLINE_CURVE_WITH_KNOTS('',3,(#15866,#15867,#15868,#15869),
 .UNSPECIFIED.,.F.,.F.,(4,4),(9.91798263530139,10.2237206759544),
 .UNSPECIFIED.);
#665=B_SPLINE_CURVE_WITH_KNOTS('',3,(#15871,#15872,#15873,#15874,#15875,
#15876,#15877,#15878,#15879,#15880,#15881,#15882,#15883,#15884,#15885,#15886,
#15887,#15888,#15889,#15890,#15891,#15892,#15893,#15894,#15895,#15896,#15897,
#15898),.UNSPECIFIED.,.F.,.F.,(4,3,3,3,3,3,3,3,3,4),(0.,0.023807020713713,
0.039085080816122,0.0628703378723092,0.0651394887354207,0.0780750047750988,
0.101981498769656,0.114997221725907,0.138748569029605,0.151942344104828),
 .UNSPECIFIED.);
#666=B_SPLINE_CURVE_WITH_KNOTS('',3,(#15902,#15903,#15904,#15905,#15906,
#15907,#15908,#15909,#15910,#15911,#15912,#15913,#15914,#15915,#15916,#15917,
#15918,#15919,#15920,#15921,#15922,#15923,#15924,#15925,#15926,#15927,#15928,
#15929),.UNSPECIFIED.,.F.,.F.,(4,3,3,3,3,3,3,3,3,4),(0.,0.0238098191818892,
0.0391006681981376,0.0628849269680955,0.0651459659463291,0.0780999162396042,
0.102007524384594,0.115011225379555,0.138759376430353,0.151943200125079),
 .UNSPECIFIED.);
#667=B_SPLINE_CURVE_WITH_KNOTS('',3,(#15931,#15932,#15933,#15934),
 .UNSPECIFIED.,.F.,.F.,(4,4),(2.85486020485948E-5,0.305707210239178),
 .UNSPECIFIED.);
#668=B_SPLINE_CURVE_WITH_KNOTS('',3,(#15944,#15945,#15946,#15947,#15948,
#15949),.UNSPECIFIED.,.F.,.F.,(4,2,4),(-0.606446248197249,-0.303383959626182,
-6.4365448350312E-5),.UNSPECIFIED.);
#669=B_SPLINE_CURVE_WITH_KNOTS('',3,(#15951,#15952,#15953,#15954,#15955,
#15956),.UNSPECIFIED.,.F.,.F.,(4,2,4),(-0.60675170080159,-0.303384112192838,
-0.000369837888147484),.UNSPECIFIED.);
#670=B_SPLINE_CURVE_WITH_KNOTS('',3,(#15958,#15959,#15960,#15961,#15962,
#15963,#15964,#15965,#15966,#15967,#15968,#15969,#15970,#15971,#15972,#15973,
#15974,#15975,#15976,#15977,#15978,#15979,#15980,#15981,#15982,#15983,#15984,
#15985),.UNSPECIFIED.,.F.,.F.,(4,3,3,3,3,3,3,3,3,4),(-0.152162866344201,
-0.128411131698784,-0.115108013904405,-0.0911850729173883,-0.0780642464630149,
-0.0652023242402653,-0.0414053499882389,-0.0390151293250392,-0.0152279490549848,
0.),.UNSPECIFIED.);
#671=B_SPLINE_CURVE_WITH_KNOTS('',3,(#15988,#15989,#15990,#15991,#15992,
#15993,#15994,#15995,#15996,#15997,#15998,#15999,#16000,#16001,#16002,#16003,
#16004,#16005,#16006,#16007,#16008,#16009,#16010,#16011,#16012,#16013,#16014,
#16015),.UNSPECIFIED.,.F.,.F.,(4,3,3,3,3,3,3,3,3,4),(-0.152171297476962,
-0.128400300768352,-0.115247520946962,-0.0914735511738372,-0.0869860114952295,
-0.0783112904282795,-0.0544025203706761,-0.0391699941254272,-0.015391764586027,
0.),.UNSPECIFIED.);
#672=B_SPLINE_CURVE_WITH_KNOTS('',3,(#16032,#16033,#16034,#16035),
 .UNSPECIFIED.,.F.,.F.,(4,4),(-3.45733745322815,-0.757207059295936),
 .UNSPECIFIED.);
#673=B_SPLINE_CURVE_WITH_KNOTS('',3,(#16053,#16054,#16055,#16056),
 .UNSPECIFIED.,.F.,.F.,(4,4),(-0.557056952888827,-0.283259008618247),
 .UNSPECIFIED.);
#674=B_SPLINE_CURVE_WITH_KNOTS('',3,(#16057,#16058,#16059,#16060),
 .UNSPECIFIED.,.F.,.F.,(4,4),(-0.618164468641375,-0.0110156167597059),
 .UNSPECIFIED.);
#675=B_SPLINE_CURVE_WITH_KNOTS('',3,(#16102,#16103,#16104,#16105),
 .UNSPECIFIED.,.F.,.F.,(4,4),(0.283259011433088,0.551788488929761),
 .UNSPECIFIED.);
#676=B_SPLINE_CURVE_WITH_KNOTS('',3,(#16109,#16110,#16111,#16112),
 .UNSPECIFIED.,.F.,.F.,(4,4),(10.1507419987596,10.419271481025),
 .UNSPECIFIED.);
#677=B_SPLINE_CURVE_WITH_KNOTS('',3,(#16147,#16148,#16149,#16150),
 .UNSPECIFIED.,.F.,.F.,(4,4),(0.0110156167597055,0.618164468641375),
 .UNSPECIFIED.);
#678=B_SPLINE_CURVE_WITH_KNOTS('',3,(#16151,#16152,#16153,#16154),
 .UNSPECIFIED.,.F.,.F.,(4,4),(-10.419271481025,-10.1454735367545),
 .UNSPECIFIED.);
#679=B_SPLINE_CURVE_WITH_KNOTS('',3,(#16157,#16158,#16159,#16160,#16161,
#16162),.UNSPECIFIED.,.F.,.F.,(4,2,4),(-0.606211482799139,-0.303431960476852,
-9.19895310989571E-5),.UNSPECIFIED.);
#680=B_SPLINE_CURVE_WITH_KNOTS('',3,(#16164,#16165,#16166,#16167,#16168,
#16169,#16170,#16171,#16172,#16173,#16174,#16175,#16176,#16177,#16178,#16179,
#16180,#16181,#16182,#16183,#16184,#16185,#16186,#16187,#16188,#16189,#16190,
#16191),.UNSPECIFIED.,.F.,.F.,(4,3,3,3,3,3,3,3,3,4),(-0.152283340966725,
-0.128554242174982,-0.115196092098682,-0.0912819860997417,-0.0781117853096875,
-0.0652755629514801,-0.0414857317972147,-0.039051434275634,-0.0152612146291672,
0.),.UNSPECIFIED.);
#681=B_SPLINE_CURVE_WITH_KNOTS('',3,(#16195,#16196,#16197,#16198,#16199,
#16200,#16201,#16202,#16203,#16204,#16205,#16206,#16207,#16208,#16209,#16210,
#16211,#16212,#16213,#16214,#16215,#16216,#16217,#16218,#16219,#16220,#16221,
#16222),.UNSPECIFIED.,.F.,.F.,(4,3,3,3,3,3,3,3,3,4),(-0.152285570909379,
-0.128511627155755,-0.115232904621082,-0.0914664612111958,-0.0870286654075453,
-0.0781769338106538,-0.0542752301960614,-0.039092246575741,-0.0153386136911565,
0.),.UNSPECIFIED.);
#682=B_SPLINE_CURVE_WITH_KNOTS('',3,(#16223,#16224,#16225,#16226,#16227,
#16228),.UNSPECIFIED.,.F.,.F.,(4,2,4),(-0.606773318344362,-0.303431998667662,
-0.000653802131222458),.UNSPECIFIED.);
#683=B_SPLINE_CURVE_WITH_KNOTS('',3,(#16245,#16246,#16247,#16248),
 .UNSPECIFIED.,.F.,.F.,(4,4),(-7.05313168653828,-3.6572084986735),
 .UNSPECIFIED.);
#684=B_SPLINE_CURVE_WITH_KNOTS('',3,(#16269,#16270,#16271,#16272),
 .UNSPECIFIED.,.F.,.F.,(4,4),(3.65450559744172,7.0548588409572),
 .UNSPECIFIED.);
#685=B_SPLINE_CURVE_WITH_KNOTS('',3,(#16274,#16275,#16276,#16277),
 .UNSPECIFIED.,.F.,.F.,(4,4),(3.64767164868607,7.04802489220155),
 .UNSPECIFIED.);
#686=B_SPLINE_CURVE_WITH_KNOTS('',3,(#16298,#16299,#16300,#16301),
 .UNSPECIFIED.,.F.,.F.,(4,4),(-7.04532199096977,-3.64939880310499),
 .UNSPECIFIED.);
#687=B_SPLINE_CURVE_WITH_KNOTS('',3,(#16320,#16321,#16322,#16323,#16324,
#16325),.UNSPECIFIED.,.F.,.F.,(4,2,4),(-0.606200453641641,-0.30343602424441,
-9.0120313562092E-5),.UNSPECIFIED.);
#688=B_SPLINE_CURVE_WITH_KNOTS('',3,(#16327,#16328,#16329,#16330,#16331,
#16332,#16333,#16334,#16335,#16336,#16337,#16338,#16339,#16340,#16341,#16342,
#16343,#16344,#16345,#16346,#16347,#16348,#16349,#16350,#16351,#16352,#16353,
#16354),.UNSPECIFIED.,.F.,.F.,(4,3,3,3,3,3,3,3,3,4),(-0.152277688086818,
-0.128551334178815,-0.115197577176818,-0.0912856014461669,-0.0781191417238373,
-0.0652765169533013,-0.0414883027365163,-0.0390570310290822,-0.0152653090895913,
0.),.UNSPECIFIED.);
#689=B_SPLINE_CURVE_WITH_KNOTS('',3,(#16356,#16357,#16358,#16359,#16360,
#16361),.UNSPECIFIED.,.F.,.F.,(4,2,4),(-0.60678286609787,-0.303436074842897,
-0.000672492961417026),.UNSPECIFIED.);
#690=B_SPLINE_CURVE_WITH_KNOTS('',3,(#16378,#16379,#16380,#16381),
 .UNSPECIFIED.,.F.,.F.,(4,4),(-9.65082888146972,-7.25285594219682),
 .UNSPECIFIED.);
#691=B_SPLINE_CURVE_WITH_KNOTS('',3,(#16402,#16403,#16404,#16405),
 .UNSPECIFIED.,.F.,.F.,(4,4),(7.25489642332205,7.94751235889625),
 .UNSPECIFIED.);
#692=B_SPLINE_CURVE_WITH_KNOTS('',3,(#16406,#16407,#16408,#16409),
 .UNSPECIFIED.,.F.,.F.,(4,4),(8.17787511801303,9.65708648657758),
 .UNSPECIFIED.);
#693=B_SPLINE_CURVE_WITH_KNOTS('',3,(#16429,#16430,#16431,#16432,#16433,
#16434),.UNSPECIFIED.,.F.,.F.,(4,2,4),(-0.607007797795788,-0.303636495504298,
-0.000571323176327465),.UNSPECIFIED.);
#694=B_SPLINE_CURVE_WITH_KNOTS('',3,(#16436,#16437,#16438,#16439,#16440,
#16441,#16442,#16443,#16444,#16445,#16446,#16447,#16448,#16449,#16450,#16451,
#16452,#16453,#16454,#16455,#16456,#16457,#16458,#16459,#16460,#16461,#16462,
#16463),.UNSPECIFIED.,.F.,.F.,(4,3,3,3,3,3,3,3,3,4),(-0.152184339020145,
-0.128410461444444,-0.115096394428865,-0.0911692948751363,-0.0780261759644403,
-0.0651939085034322,-0.0413932235702045,-0.0389860720679279,-0.0151971168406065,
0.),.UNSPECIFIED.);
#695=B_SPLINE_CURVE_WITH_KNOTS('',3,(#16467,#16468,#16469,#16470,#16471,
#16472,#16473,#16474,#16475,#16476,#16477,#16478,#16479,#16480,#16481,#16482,
#16483,#16484,#16485,#16486,#16487,#16488,#16489,#16490,#16491,#16492,#16493,
#16494),.UNSPECIFIED.,.F.,.F.,(4,3,3,3,3,3,3,3,3,4),(-0.15219777746951,
-0.128424216118147,-0.115318679085322,-0.0915406112613293,-0.0870190514838729,
-0.0784197287877601,-0.0545085386658457,-0.0392329067084975,-0.0154317870320417,
0.),.UNSPECIFIED.);
#696=B_SPLINE_CURVE_WITH_KNOTS('',3,(#16495,#16496,#16497,#16498,#16499,
#16500),.UNSPECIFIED.,.F.,.F.,(4,2,4),(-0.606706256981509,-0.303636876939173,
-0.00026974181288697),.UNSPECIFIED.);
#697=B_SPLINE_CURVE_WITH_KNOTS('',3,(#16518,#16519,#16520,#16521),
 .UNSPECIFIED.,.F.,.F.,(4,4),(0.0112334529114386,0.618489359031386),
 .UNSPECIFIED.);
#698=B_SPLINE_CURVE_WITH_KNOTS('',3,(#16522,#16523,#16524,#16525),
 .UNSPECIFIED.,.F.,.F.,(4,4),(-10.4271318523291,-9.85085636625011),
 .UNSPECIFIED.);
#699=B_SPLINE_CURVE_WITH_KNOTS('',3,(#16548,#16549,#16550,#16551),
 .UNSPECIFIED.,.F.,.F.,(4,4),(9.85750350611301,10.4271318523291),
 .UNSPECIFIED.);
#700=B_SPLINE_CURVE_WITH_KNOTS('',3,(#16555,#16556,#16557,#16558),
 .UNSPECIFIED.,.F.,.F.,(4,4),(0.27539863731415,0.845026983530265),
 .UNSPECIFIED.);
#701=B_SPLINE_CURVE_WITH_KNOTS('',3,(#16576,#16577,#16578,#16579),
 .UNSPECIFIED.,.F.,.F.,(4,4),(-0.851674123393175,-0.27539863731415),
 .UNSPECIFIED.);
#702=B_SPLINE_CURVE_WITH_KNOTS('',3,(#16580,#16581,#16582,#16583),
 .UNSPECIFIED.,.F.,.F.,(4,4),(-0.618489359031386,-0.0112334529114389),
 .UNSPECIFIED.);
#703=B_SPLINE_CURVE_WITH_KNOTS('',3,(#16663,#16664,#16665,#16666),
 .UNSPECIFIED.,.F.,.F.,(4,4),(0.0112755522169305,0.618164468641375),
 .UNSPECIFIED.);
#704=B_SPLINE_CURVE_WITH_KNOTS('',3,(#16687,#16688,#16689,#16690),
 .UNSPECIFIED.,.F.,.F.,(4,4),(-0.618164468641375,-0.0112755522169305),
 .UNSPECIFIED.);
#705=B_SPLINE_CURVE_WITH_KNOTS('',3,(#16776,#16777,#16778,#16779),
 .UNSPECIFIED.,.F.,.F.,(4,4),(5.55111512312578E-17,0.618489359031386),
 .UNSPECIFIED.);
#706=B_SPLINE_CURVE_WITH_KNOTS('',3,(#16780,#16781,#16782,#16783),
 .UNSPECIFIED.,.F.,.F.,(4,4),(-0.618489359031386,-0.00110654915602034),
 .UNSPECIFIED.);
#707=B_SPLINE_CURVE_WITH_KNOTS('',3,(#16819,#16820,#16821,#16822,#16823),
 .UNSPECIFIED.,.F.,.F.,(4,1,4),(-10.4271318523291,-4.63063308449434,-0.283259008618247),
 .UNSPECIFIED.);
#708=B_SPLINE_CURVE_WITH_KNOTS('',3,(#16824,#16825,#16826,#16827,#16828),
 .UNSPECIFIED.,.F.,.F.,(4,1,4),(0.283259011433087,4.63063308449434,10.4271318523291),
 .UNSPECIFIED.);
#709=B_SPLINE_CURVE_WITH_KNOTS('',3,(#16849,#16850,#16851,#16852),
 .UNSPECIFIED.,.F.,.F.,(4,4),(0.000779732613545348,0.618164468641375),
 .UNSPECIFIED.);
#710=B_SPLINE_CURVE_WITH_KNOTS('',3,(#16853,#16854,#16855,#16856),
 .UNSPECIFIED.,.F.,.F.,(4,4),(-0.618164468641375,-4.9439619065339E-17),
 .UNSPECIFIED.);
#711=B_SPLINE_CURVE_WITH_KNOTS('',3,(#16877,#16878,#16879,#16880),
 .UNSPECIFIED.,.F.,.F.,(4,4),(3.0964814046186E-16,0.618164468641375),
 .UNSPECIFIED.);
#712=B_SPLINE_CURVE_WITH_KNOTS('',3,(#16881,#16882,#16883,#16884),
 .UNSPECIFIED.,.F.,.F.,(4,4),(-0.618164468641375,-0.0007797326135453),
 .UNSPECIFIED.);
#713=B_SPLINE_CURVE_WITH_KNOTS('',3,(#16910,#16911,#16912,#16913,#16914),
 .UNSPECIFIED.,.F.,.F.,(4,1,4),(-10.419271481025,-4.62277271319024,-0.27539863731415),
 .UNSPECIFIED.);
#714=B_SPLINE_CURVE_WITH_KNOTS('',3,(#16915,#16916,#16917,#16918,#16919),
 .UNSPECIFIED.,.F.,.F.,(4,1,4),(0.27539863731415,4.62277271319024,10.419271481025),
 .UNSPECIFIED.);
#715=B_SPLINE_CURVE_WITH_KNOTS('',3,(#16940,#16941,#16942,#16943),
 .UNSPECIFIED.,.F.,.F.,(4,4),(0.00110654915602046,0.618489359031386),
 .UNSPECIFIED.);
#716=B_SPLINE_CURVE_WITH_KNOTS('',3,(#16944,#16945,#16946,#16947),
 .UNSPECIFIED.,.F.,.F.,(4,4),(-0.618489359031386,6.93889390390723E-18),
 .UNSPECIFIED.);
#1196=PLANE('',#10270);
#1197=PLANE('',#10287);
#1198=PLANE('',#10292);
#1199=PLANE('',#10298);
#1200=PLANE('',#10299);
#1201=PLANE('',#10300);
#1202=PLANE('',#10301);
#1203=PLANE('',#10302);
#1204=PLANE('',#10303);
#1205=PLANE('',#10304);
#1206=PLANE('',#10305);
#1207=PLANE('',#10307);
#1208=PLANE('',#10309);
#1209=PLANE('',#10310);
#1210=PLANE('',#10311);
#1211=PLANE('',#10312);
#1212=PLANE('',#10313);
#1213=PLANE('',#10314);
#1214=PLANE('',#10315);
#1215=PLANE('',#10316);
#1216=PLANE('',#10317);
#1217=PLANE('',#10318);
#1218=PLANE('',#10319);
#1219=PLANE('',#10323);
#1220=PLANE('',#10325);
#1221=PLANE('',#10326);
#1222=PLANE('',#10327);
#1223=PLANE('',#10328);
#1224=PLANE('',#10329);
#1225=PLANE('',#10330);
#1226=PLANE('',#10332);
#1227=PLANE('',#10349);
#1228=PLANE('',#10368);
#1229=PLANE('',#10369);
#1230=PLANE('',#10370);
#1529=FACE_OUTER_BOUND('',#2097,.T.);
#1530=FACE_OUTER_BOUND('',#2098,.T.);
#1531=FACE_OUTER_BOUND('',#2099,.T.);
#1532=FACE_OUTER_BOUND('',#2100,.T.);
#1533=FACE_OUTER_BOUND('',#2101,.T.);
#1534=FACE_OUTER_BOUND('',#2102,.T.);
#1535=FACE_OUTER_BOUND('',#2103,.T.);
#1536=FACE_OUTER_BOUND('',#2107,.T.);
#1537=FACE_OUTER_BOUND('',#2108,.T.);
#1538=FACE_OUTER_BOUND('',#2109,.T.);
#1539=FACE_OUTER_BOUND('',#2110,.T.);
#1540=FACE_OUTER_BOUND('',#2111,.T.);
#1541=FACE_OUTER_BOUND('',#2112,.T.);
#1542=FACE_OUTER_BOUND('',#2114,.T.);
#1543=FACE_OUTER_BOUND('',#2115,.T.);
#1544=FACE_OUTER_BOUND('',#2117,.T.);
#1545=FACE_OUTER_BOUND('',#2118,.T.);
#1546=FACE_OUTER_BOUND('',#2119,.T.);
#1547=FACE_OUTER_BOUND('',#2120,.T.);
#1548=FACE_OUTER_BOUND('',#2121,.T.);
#1549=FACE_OUTER_BOUND('',#2122,.T.);
#1550=FACE_OUTER_BOUND('',#2123,.T.);
#1551=FACE_OUTER_BOUND('',#2124,.T.);
#1552=FACE_OUTER_BOUND('',#2125,.T.);
#1553=FACE_OUTER_BOUND('',#2126,.T.);
#1554=FACE_OUTER_BOUND('',#2128,.T.);
#1555=FACE_OUTER_BOUND('',#2130,.T.);
#1556=FACE_OUTER_BOUND('',#2131,.T.);
#1557=FACE_OUTER_BOUND('',#2132,.T.);
#1558=FACE_OUTER_BOUND('',#2133,.T.);
#1559=FACE_OUTER_BOUND('',#2134,.T.);
#1560=FACE_OUTER_BOUND('',#2135,.T.);
#1561=FACE_OUTER_BOUND('',#2136,.T.);
#1562=FACE_OUTER_BOUND('',#2137,.T.);
#1563=FACE_OUTER_BOUND('',#2138,.T.);
#1564=FACE_OUTER_BOUND('',#2139,.T.);
#1565=FACE_OUTER_BOUND('',#2140,.T.);
#1566=FACE_OUTER_BOUND('',#2142,.T.);
#1567=FACE_OUTER_BOUND('',#2143,.T.);
#1568=FACE_OUTER_BOUND('',#2144,.T.);
#1569=FACE_OUTER_BOUND('',#2145,.T.);
#1570=FACE_OUTER_BOUND('',#2146,.T.);
#1571=FACE_OUTER_BOUND('',#2147,.T.);
#1572=FACE_OUTER_BOUND('',#2148,.T.);
#1573=FACE_OUTER_BOUND('',#2149,.T.);
#1574=FACE_OUTER_BOUND('',#2150,.T.);
#1575=FACE_OUTER_BOUND('',#2151,.T.);
#1576=FACE_OUTER_BOUND('',#2152,.T.);
#1577=FACE_OUTER_BOUND('',#2153,.T.);
#1578=FACE_OUTER_BOUND('',#2154,.T.);
#1579=FACE_OUTER_BOUND('',#2155,.T.);
#1580=FACE_OUTER_BOUND('',#2156,.T.);
#1581=FACE_OUTER_BOUND('',#2157,.T.);
#1582=FACE_OUTER_BOUND('',#2158,.T.);
#1583=FACE_OUTER_BOUND('',#2159,.T.);
#1584=FACE_OUTER_BOUND('',#2160,.T.);
#1585=FACE_OUTER_BOUND('',#2161,.T.);
#1586=FACE_OUTER_BOUND('',#2165,.T.);
#1587=FACE_OUTER_BOUND('',#2166,.T.);
#1588=FACE_OUTER_BOUND('',#2167,.T.);
#1589=FACE_OUTER_BOUND('',#2168,.T.);
#1590=FACE_OUTER_BOUND('',#2169,.T.);
#1591=FACE_OUTER_BOUND('',#2170,.T.);
#1592=FACE_OUTER_BOUND('',#2171,.T.);
#1593=FACE_OUTER_BOUND('',#2172,.T.);
#1594=FACE_OUTER_BOUND('',#2173,.T.);
#1595=FACE_OUTER_BOUND('',#2174,.T.);
#1596=FACE_OUTER_BOUND('',#2175,.T.);
#1597=FACE_OUTER_BOUND('',#2176,.T.);
#1598=FACE_OUTER_BOUND('',#2177,.T.);
#1599=FACE_OUTER_BOUND('',#2178,.T.);
#1600=FACE_OUTER_BOUND('',#2179,.T.);
#1601=FACE_OUTER_BOUND('',#2180,.T.);
#1602=FACE_OUTER_BOUND('',#2181,.T.);
#1603=FACE_OUTER_BOUND('',#2182,.T.);
#1604=FACE_OUTER_BOUND('',#2183,.T.);
#1605=FACE_OUTER_BOUND('',#2184,.T.);
#1606=FACE_OUTER_BOUND('',#2185,.T.);
#1607=FACE_OUTER_BOUND('',#2186,.T.);
#1608=FACE_OUTER_BOUND('',#2187,.T.);
#1609=FACE_OUTER_BOUND('',#2188,.T.);
#1610=FACE_OUTER_BOUND('',#2189,.T.);
#1611=FACE_OUTER_BOUND('',#2190,.T.);
#1612=FACE_OUTER_BOUND('',#2191,.T.);
#1613=FACE_OUTER_BOUND('',#2192,.T.);
#1614=FACE_OUTER_BOUND('',#2193,.T.);
#1615=FACE_OUTER_BOUND('',#2194,.T.);
#1616=FACE_OUTER_BOUND('',#2195,.T.);
#1617=FACE_OUTER_BOUND('',#2196,.T.);
#1618=FACE_OUTER_BOUND('',#2197,.T.);
#1619=FACE_OUTER_BOUND('',#2198,.T.);
#1620=FACE_OUTER_BOUND('',#2205,.T.);
#1621=FACE_OUTER_BOUND('',#2206,.T.);
#2097=EDGE_LOOP('',(#7497,#7498));
#2098=EDGE_LOOP('',(#7499,#7500));
#2099=EDGE_LOOP('',(#7501,#7502));
#2100=EDGE_LOOP('',(#7503,#7504));
#2101=EDGE_LOOP('',(#7505,#7506,#7507,#7508,#7509,#7510));
#2102=EDGE_LOOP('',(#7511,#7512,#7513,#7514,#7515,#7516));
#2103=EDGE_LOOP('',(#7517,#7518,#7519,#7520,#7521,#7522,#7523,#7524));
#2104=EDGE_LOOP('',(#7525));
#2105=EDGE_LOOP('',(#7526));
#2106=EDGE_LOOP('',(#7527));
#2107=EDGE_LOOP('',(#7528,#7529,#7530,#7531));
#2108=EDGE_LOOP('',(#7532,#7533,#7534,#7535));
#2109=EDGE_LOOP('',(#7536,#7537,#7538,#7539));
#2110=EDGE_LOOP('',(#7540,#7541,#7542,#7543));
#2111=EDGE_LOOP('',(#7544,#7545,#7546,#7547));
#2112=EDGE_LOOP('',(#7548));
#2113=EDGE_LOOP('',(#7549));
#2114=EDGE_LOOP('',(#7550,#7551,#7552,#7553));
#2115=EDGE_LOOP('',(#7554));
#2116=EDGE_LOOP('',(#7555));
#2117=EDGE_LOOP('',(#7556,#7557,#7558,#7559));
#2118=EDGE_LOOP('',(#7560,#7561,#7562,#7563));
#2119=EDGE_LOOP('',(#7564,#7565,#7566,#7567));
#2120=EDGE_LOOP('',(#7568,#7569,#7570,#7571));
#2121=EDGE_LOOP('',(#7572,#7573,#7574,#7575));
#2122=EDGE_LOOP('',(#7576,#7577,#7578,#7579));
#2123=EDGE_LOOP('',(#7580,#7581,#7582,#7583));
#2124=EDGE_LOOP('',(#7584,#7585,#7586,#7587));
#2125=EDGE_LOOP('',(#7588,#7589,#7590,#7591));
#2126=EDGE_LOOP('',(#7592));
#2127=EDGE_LOOP('',(#7593));
#2128=EDGE_LOOP('',(#7594));
#2129=EDGE_LOOP('',(#7595));
#2130=EDGE_LOOP('',(#7596,#7597,#7598,#7599));
#2131=EDGE_LOOP('',(#7600,#7601,#7602,#7603));
#2132=EDGE_LOOP('',(#7604,#7605,#7606,#7607));
#2133=EDGE_LOOP('',(#7608,#7609,#7610,#7611));
#2134=EDGE_LOOP('',(#7612,#7613,#7614,#7615));
#2135=EDGE_LOOP('',(#7616,#7617,#7618,#7619,#7620,#7621));
#2136=EDGE_LOOP('',(#7622,#7623,#7624,#7625,#7626,#7627,#7628,#7629,#7630,
#7631));
#2137=EDGE_LOOP('',(#7632,#7633,#7634,#7635,#7636,#7637,#7638,#7639,#7640,
#7641));
#2138=EDGE_LOOP('',(#7642,#7643,#7644,#7645,#7646,#7647,#7648,#7649,#7650,
#7651));
#2139=EDGE_LOOP('',(#7652,#7653,#7654,#7655,#7656,#7657,#7658,#7659));
#2140=EDGE_LOOP('',(#7660,#7661,#7662,#7663,#7664,#7665,#7666,#7667,#7668,
#7669,#7670,#7671,#7672,#7673,#7674,#7675,#7676,#7677,#7678,#7679,#7680,
#7681,#7682,#7683,#7684,#7685,#7686,#7687,#7688,#7689,#7690,#7691,#7692,
#7693,#7694,#7695,#7696,#7697,#7698,#7699,#7700,#7701));
#2141=EDGE_LOOP('',(#7702,#7703,#7704,#7705,#7706,#7707));
#2142=EDGE_LOOP('',(#7708,#7709,#7710,#7711));
#2143=EDGE_LOOP('',(#7712,#7713,#7714,#7715));
#2144=EDGE_LOOP('',(#7716,#7717,#7718,#7719,#7720,#7721));
#2145=EDGE_LOOP('',(#7722,#7723,#7724,#7725));
#2146=EDGE_LOOP('',(#7726,#7727,#7728,#7729));
#2147=EDGE_LOOP('',(#7730,#7731,#7732,#7733,#7734,#7735));
#2148=EDGE_LOOP('',(#7736,#7737,#7738,#7739));
#2149=EDGE_LOOP('',(#7740,#7741,#7742,#7743));
#2150=EDGE_LOOP('',(#7744,#7745,#7746,#7747));
#2151=EDGE_LOOP('',(#7748,#7749,#7750,#7751));
#2152=EDGE_LOOP('',(#7752,#7753,#7754,#7755,#7756,#7757,#7758,#7759,#7760,
#7761));
#2153=EDGE_LOOP('',(#7762,#7763,#7764,#7765));
#2154=EDGE_LOOP('',(#7766,#7767,#7768,#7769));
#2155=EDGE_LOOP('',(#7770,#7771,#7772,#7773));
#2156=EDGE_LOOP('',(#7774,#7775,#7776,#7777));
#2157=EDGE_LOOP('',(#7778,#7779,#7780,#7781));
#2158=EDGE_LOOP('',(#7782,#7783,#7784,#7785,#7786,#7787,#7788,#7789,#7790,
#7791));
#2159=EDGE_LOOP('',(#7792,#7793,#7794,#7795));
#2160=EDGE_LOOP('',(#7796,#7797,#7798,#7799,#7800,#7801));
#2161=EDGE_LOOP('',(#7802,#7803,#7804,#7805,#7806,#7807,#7808,#7809));
#2162=EDGE_LOOP('',(#7810));
#2163=EDGE_LOOP('',(#7811));
#2164=EDGE_LOOP('',(#7812));
#2165=EDGE_LOOP('',(#7813,#7814,#7815,#7816));
#2166=EDGE_LOOP('',(#7817,#7818,#7819,#7820,#7821,#7822,#7823,#7824,#7825,
#7826));
#2167=EDGE_LOOP('',(#7827,#7828,#7829,#7830));
#2168=EDGE_LOOP('',(#7831,#7832,#7833,#7834));
#2169=EDGE_LOOP('',(#7835,#7836,#7837,#7838));
#2170=EDGE_LOOP('',(#7839,#7840,#7841,#7842));
#2171=EDGE_LOOP('',(#7843,#7844,#7845,#7846));
#2172=EDGE_LOOP('',(#7847,#7848,#7849));
#2173=EDGE_LOOP('',(#7850,#7851,#7852));
#2174=EDGE_LOOP('',(#7853,#7854,#7855));
#2175=EDGE_LOOP('',(#7856,#7857,#7858,#7859));
#2176=EDGE_LOOP('',(#7860,#7861,#7862,#7863));
#2177=EDGE_LOOP('',(#7864,#7865,#7866));
#2178=EDGE_LOOP('',(#7867,#7868,#7869,#7870));
#2179=EDGE_LOOP('',(#7871,#7872,#7873,#7874));
#2180=EDGE_LOOP('',(#7875,#7876,#7877,#7878));
#2181=EDGE_LOOP('',(#7879,#7880,#7881,#7882));
#2182=EDGE_LOOP('',(#7883,#7884,#7885,#7886));
#2183=EDGE_LOOP('',(#7887,#7888,#7889,#7890));
#2184=EDGE_LOOP('',(#7891,#7892,#7893));
#2185=EDGE_LOOP('',(#7894,#7895,#7896));
#2186=EDGE_LOOP('',(#7897,#7898,#7899));
#2187=EDGE_LOOP('',(#7900,#7901,#7902,#7903));
#2188=EDGE_LOOP('',(#7904,#7905,#7906,#7907));
#2189=EDGE_LOOP('',(#7908,#7909,#7910));
#2190=EDGE_LOOP('',(#7911,#7912,#7913,#7914));
#2191=EDGE_LOOP('',(#7915,#7916,#7917,#7918));
#2192=EDGE_LOOP('',(#7919,#7920,#7921,#7922));
#2193=EDGE_LOOP('',(#7923,#7924,#7925,#7926));
#2194=EDGE_LOOP('',(#7927,#7928,#7929,#7930));
#2195=EDGE_LOOP('',(#7931,#7932,#7933,#7934));
#2196=EDGE_LOOP('',(#7935,#7936,#7937,#7938));
#2197=EDGE_LOOP('',(#7939,#7940,#7941,#7942,#7943,#7944,#7945,#7946));
#2198=EDGE_LOOP('',(#7947,#7948,#7949,#7950));
#2199=EDGE_LOOP('',(#7951));
#2200=EDGE_LOOP('',(#7952));
#2201=EDGE_LOOP('',(#7953));
#2202=EDGE_LOOP('',(#7954));
#2203=EDGE_LOOP('',(#7955));
#2204=EDGE_LOOP('',(#7956));
#2205=EDGE_LOOP('',(#7957,#7958,#7959,#7960));
#2206=EDGE_LOOP('',(#7961,#7962,#7963,#7964));
#2739=LINE('',#15233,#3327);
#2740=LINE('',#15235,#3328);
#2741=LINE('',#15249,#3329);
#2742=LINE('',#15254,#3330);
#2743=LINE('',#15260,#3331);
#2744=LINE('',#15265,#3332);
#2745=LINE('',#15270,#3333);
#2746=LINE('',#15279,#3334);
#2747=LINE('',#15286,#3335);
#2748=LINE('',#15290,#3336);
#2749=LINE('',#15295,#3337);
#2750=LINE('',#15297,#3338);
#2751=LINE('',#15299,#3339);
#2752=LINE('',#15300,#3340);
#2753=LINE('',#15304,#3341);
#2754=LINE('',#15306,#3342);
#2755=LINE('',#15308,#3343);
#2756=LINE('',#15309,#3344);
#2757=LINE('',#15313,#3345);
#2758=LINE('',#15315,#3346);
#2759=LINE('',#15317,#3347);
#2760=LINE('',#15318,#3348);
#2761=LINE('',#15322,#3349);
#2762=LINE('',#15324,#3350);
#2763=LINE('',#15326,#3351);
#2764=LINE('',#15327,#3352);
#2765=LINE('',#15331,#3353);
#2766=LINE('',#15333,#3354);
#2767=LINE('',#15335,#3355);
#2768=LINE('',#15336,#3356);
#2769=LINE('',#15340,#3357);
#2770=LINE('',#15342,#3358);
#2771=LINE('',#15344,#3359);
#2772=LINE('',#15345,#3360);
#2773=LINE('',#15349,#3361);
#2774=LINE('',#15351,#3362);
#2775=LINE('',#15353,#3363);
#2776=LINE('',#15354,#3364);
#2777=LINE('',#15362,#3365);
#2778=LINE('',#15363,#3366);
#2779=LINE('',#15365,#3367);
#2780=LINE('',#15366,#3368);
#2781=LINE('',#15368,#3369);
#2782=LINE('',#15369,#3370);
#2783=LINE('',#15372,#3371);
#2784=LINE('',#15374,#3372);
#2785=LINE('',#15375,#3373);
#2786=LINE('',#15378,#3374);
#2787=LINE('',#15380,#3375);
#2788=LINE('',#15381,#3376);
#2789=LINE('',#15385,#3377);
#2790=LINE('',#15429,#3378);
#2791=LINE('',#15472,#3379);
#2792=LINE('',#15475,#3380);
#2793=LINE('',#15513,#3381);
#2794=LINE('',#15550,#3382);
#2795=LINE('',#15553,#3383);
#2796=LINE('',#15561,#3384);
#2797=LINE('',#15598,#3385);
#2798=LINE('',#15601,#3386);
#2799=LINE('',#15608,#3387);
#2800=LINE('',#15614,#3388);
#2801=LINE('',#15625,#3389);
#2802=LINE('',#15634,#3390);
#2803=LINE('',#15640,#3391);
#2804=LINE('',#15675,#3392);
#2805=LINE('',#15746,#3393);
#2806=LINE('',#15816,#3394);
#2807=LINE('',#15848,#3395);
#2808=LINE('',#15854,#3396);
#2809=LINE('',#15863,#3397);
#2810=LINE('',#15900,#3398);
#2811=LINE('',#15935,#3399);
#2812=LINE('',#15937,#3400);
#2813=LINE('',#15941,#3401);
#2814=LINE('',#15987,#3402);
#2815=LINE('',#16113,#3403);
#2816=LINE('',#16193,#3404);
#2817=LINE('',#16355,#3405);
#2818=LINE('',#16465,#3406);
#2819=LINE('',#16554,#3407);
#2820=LINE('',#16642,#3408);
#2821=LINE('',#16754,#3409);
#2822=LINE('',#16755,#3410);
#2823=LINE('',#16792,#3411);
#2824=LINE('',#16793,#3412);
#3327=VECTOR('',#11451,1.);
#3328=VECTOR('',#11452,1.);
#3329=VECTOR('',#11463,0.15);
#3330=VECTOR('',#11468,0.15);
#3331=VECTOR('',#11475,0.15);
#3332=VECTOR('',#11482,0.15);
#3333=VECTOR('',#11487,0.3);
#3334=VECTOR('',#11498,0.3);
#3335=VECTOR('',#11507,0.17);
#3336=VECTOR('',#11512,0.17);
#3337=VECTOR('',#11517,1.);
#3338=VECTOR('',#11518,1.);
#3339=VECTOR('',#11519,1.);
#3340=VECTOR('',#11520,1.);
#3341=VECTOR('',#11523,1.);
#3342=VECTOR('',#11524,1.);
#3343=VECTOR('',#11525,1.);
#3344=VECTOR('',#11526,1.);
#3345=VECTOR('',#11529,1.);
#3346=VECTOR('',#11530,1.);
#3347=VECTOR('',#11531,1.);
#3348=VECTOR('',#11532,1.);
#3349=VECTOR('',#11535,1.);
#3350=VECTOR('',#11536,1.);
#3351=VECTOR('',#11537,1.);
#3352=VECTOR('',#11538,1.);
#3353=VECTOR('',#11541,1.);
#3354=VECTOR('',#11542,1.);
#3355=VECTOR('',#11543,1.);
#3356=VECTOR('',#11544,1.);
#3357=VECTOR('',#11547,1.);
#3358=VECTOR('',#11548,1.);
#3359=VECTOR('',#11549,1.);
#3360=VECTOR('',#11550,1.);
#3361=VECTOR('',#11553,1.);
#3362=VECTOR('',#11554,1.);
#3363=VECTOR('',#11555,1.);
#3364=VECTOR('',#11556,1.);
#3365=VECTOR('',#11567,1.);
#3366=VECTOR('',#11568,1.);
#3367=VECTOR('',#11571,1.);
#3368=VECTOR('',#11572,1.);
#3369=VECTOR('',#11575,1.);
#3370=VECTOR('',#11576,1.);
#3371=VECTOR('',#11579,1.);
#3372=VECTOR('',#11580,1.);
#3373=VECTOR('',#11581,1.);
#3374=VECTOR('',#11584,1.);
#3375=VECTOR('',#11585,1.);
#3376=VECTOR('',#11586,1.);
#3377=VECTOR('',#11589,1.);
#3378=VECTOR('',#11592,1.);
#3379=VECTOR('',#11593,1.);
#3380=VECTOR('',#11596,1.);
#3381=VECTOR('',#11597,1.);
#3382=VECTOR('',#11598,1.);
#3383=VECTOR('',#11601,1.);
#3384=VECTOR('',#11602,1.);
#3385=VECTOR('',#11603,1.);
#3386=VECTOR('',#11606,1.);
#3387=VECTOR('',#11607,1.);
#3388=VECTOR('',#11608,1.);
#3389=VECTOR('',#11611,1.);
#3390=VECTOR('',#11612,1.);
#3391=VECTOR('',#11613,1.);
#3392=VECTOR('',#11614,1.);
#3393=VECTOR('',#11615,1.);
#3394=VECTOR('',#11616,1.);
#3395=VECTOR('',#11617,1.);
#3396=VECTOR('',#11618,1.);
#3397=VECTOR('',#11619,1.);
#3398=VECTOR('',#11620,1.);
#3399=VECTOR('',#11621,1.);
#3400=VECTOR('',#11624,0.4);
#3401=VECTOR('',#11629,0.4);
#3402=VECTOR('',#11632,1.);
#3403=VECTOR('',#11637,1.);
#3404=VECTOR('',#11640,1.);
#3405=VECTOR('',#11645,1.);
#3406=VECTOR('',#11650,1.);
#3407=VECTOR('',#11655,1.);
#3408=VECTOR('',#11688,1.);
#3409=VECTOR('',#11717,1.);
#3410=VECTOR('',#11718,1.);
#3411=VECTOR('',#11729,1.);
#3412=VECTOR('',#11730,1.);
#3691=CIRCLE('',#10263,0.25);
#3692=CIRCLE('',#10265,0.25);
#3693=CIRCLE('',#10267,0.25);
#3694=CIRCLE('',#10269,0.25);
#3695=CIRCLE('',#10271,0.15);
#3696=CIRCLE('',#10272,0.15);
#3697=CIRCLE('',#10273,0.4);
#3698=CIRCLE('',#10275,0.15);
#3699=CIRCLE('',#10277,0.15);
#3700=CIRCLE('',#10278,0.15);
#3701=CIRCLE('',#10280,0.15);
#3702=CIRCLE('',#10281,0.15);
#3703=CIRCLE('',#10283,0.15);
#3704=CIRCLE('',#10285,0.3);
#3705=CIRCLE('',#10286,0.3);
#3706=CIRCLE('',#10288,0.17);
#3707=CIRCLE('',#10290,0.3);
#3708=CIRCLE('',#10291,0.3);
#3709=CIRCLE('',#10293,0.17);
#3710=CIRCLE('',#10295,0.17);
#3711=CIRCLE('',#10297,0.17);
#3712=CIRCLE('',#10306,0.4);
#3713=CIRCLE('',#10308,0.4);
#3714=CIRCLE('',#10322,0.4);
#3715=CIRCLE('',#10324,0.1);
#3716=CIRCLE('',#10331,0.0999999999999995);
#3717=CIRCLE('',#10333,0.1);
#3718=CIRCLE('',#10335,0.1);
#3719=CIRCLE('',#10336,0.1);
#3720=CIRCLE('',#10338,0.0999999999999999);
#3721=CIRCLE('',#10339,0.0999999999999998);
#3722=CIRCLE('',#10340,0.0999999999999998);
#3723=CIRCLE('',#10342,0.0999999999999994);
#3724=CIRCLE('',#10343,0.0999999999999993);
#3725=CIRCLE('',#10346,0.0999999999999999);
#3726=CIRCLE('',#10347,0.1);
#3727=CIRCLE('',#10351,0.3);
#3728=CIRCLE('',#10352,0.3);
#3729=CIRCLE('',#10353,0.3);
#3730=CIRCLE('',#10355,0.3);
#3731=CIRCLE('',#10356,0.3);
#3732=CIRCLE('',#10357,0.3);
#3733=CIRCLE('',#10359,0.3);
#3734=CIRCLE('',#10360,0.299999999999999);
#3735=CIRCLE('',#10361,0.3);
#3736=CIRCLE('',#10364,0.3);
#3737=CIRCLE('',#10365,0.3);
#3738=CIRCLE('',#10366,0.3);
#4239=VERTEX_POINT('',#14940);
#4240=VERTEX_POINT('',#14941);
#4241=VERTEX_POINT('',#14968);
#4242=VERTEX_POINT('',#14969);
#4243=VERTEX_POINT('',#14992);
#4244=VERTEX_POINT('',#14993);
#4245=VERTEX_POINT('',#15016);
#4246=VERTEX_POINT('',#15017);
#4247=VERTEX_POINT('',#15063);
#4248=VERTEX_POINT('',#15068);
#4249=VERTEX_POINT('',#15097);
#4250=VERTEX_POINT('',#15102);
#4251=VERTEX_POINT('',#15155);
#4252=VERTEX_POINT('',#15160);
#4253=VERTEX_POINT('',#15189);
#4254=VERTEX_POINT('',#15194);
#4255=VERTEX_POINT('',#15228);
#4256=VERTEX_POINT('',#15234);
#4257=VERTEX_POINT('',#15240);
#4258=VERTEX_POINT('',#15242);
#4259=VERTEX_POINT('',#15244);
#4260=VERTEX_POINT('',#15247);
#4261=VERTEX_POINT('',#15251);
#4262=VERTEX_POINT('',#15253);
#4263=VERTEX_POINT('',#15257);
#4264=VERTEX_POINT('',#15259);
#4265=VERTEX_POINT('',#15263);
#4266=VERTEX_POINT('',#15267);
#4267=VERTEX_POINT('',#15269);
#4268=VERTEX_POINT('',#15273);
#4269=VERTEX_POINT('',#15276);
#4270=VERTEX_POINT('',#15278);
#4271=VERTEX_POINT('',#15282);
#4272=VERTEX_POINT('',#15285);
#4273=VERTEX_POINT('',#15289);
#4274=VERTEX_POINT('',#15293);
#4275=VERTEX_POINT('',#15294);
#4276=VERTEX_POINT('',#15296);
#4277=VERTEX_POINT('',#15298);
#4278=VERTEX_POINT('',#15302);
#4279=VERTEX_POINT('',#15303);
#4280=VERTEX_POINT('',#15305);
#4281=VERTEX_POINT('',#15307);
#4282=VERTEX_POINT('',#15311);
#4283=VERTEX_POINT('',#15312);
#4284=VERTEX_POINT('',#15314);
#4285=VERTEX_POINT('',#15316);
#4286=VERTEX_POINT('',#15320);
#4287=VERTEX_POINT('',#15321);
#4288=VERTEX_POINT('',#15323);
#4289=VERTEX_POINT('',#15325);
#4290=VERTEX_POINT('',#15329);
#4291=VERTEX_POINT('',#15330);
#4292=VERTEX_POINT('',#15332);
#4293=VERTEX_POINT('',#15334);
#4294=VERTEX_POINT('',#15338);
#4295=VERTEX_POINT('',#15339);
#4296=VERTEX_POINT('',#15341);
#4297=VERTEX_POINT('',#15343);
#4298=VERTEX_POINT('',#15347);
#4299=VERTEX_POINT('',#15348);
#4300=VERTEX_POINT('',#15350);
#4301=VERTEX_POINT('',#15352);
#4302=VERTEX_POINT('',#15356);
#4303=VERTEX_POINT('',#15359);
#4304=VERTEX_POINT('',#15371);
#4305=VERTEX_POINT('',#15373);
#4306=VERTEX_POINT('',#15377);
#4307=VERTEX_POINT('',#15379);
#4308=VERTEX_POINT('',#15383);
#4309=VERTEX_POINT('',#15384);
#4310=VERTEX_POINT('',#15386);
#4311=VERTEX_POINT('',#15428);
#4312=VERTEX_POINT('',#15436);
#4313=VERTEX_POINT('',#15465);
#4314=VERTEX_POINT('',#15474);
#4315=VERTEX_POINT('',#15476);
#4316=VERTEX_POINT('',#15483);
#4317=VERTEX_POINT('',#15512);
#4318=VERTEX_POINT('',#15514);
#4319=VERTEX_POINT('',#15543);
#4320=VERTEX_POINT('',#15552);
#4321=VERTEX_POINT('',#15560);
#4322=VERTEX_POINT('',#15562);
#4323=VERTEX_POINT('',#15591);
#4324=VERTEX_POINT('',#15600);
#4325=VERTEX_POINT('',#15602);
#4326=VERTEX_POINT('',#15607);
#4327=VERTEX_POINT('',#15609);
#4328=VERTEX_POINT('',#15624);
#4329=VERTEX_POINT('',#15633);
#4330=VERTEX_POINT('',#15639);
#4331=VERTEX_POINT('',#15641);
#4332=VERTEX_POINT('',#15674);
#4333=VERTEX_POINT('',#15676);
#4334=VERTEX_POINT('',#15708);
#4335=VERTEX_POINT('',#15713);
#4336=VERTEX_POINT('',#15745);
#4337=VERTEX_POINT('',#15747);
#4338=VERTEX_POINT('',#15779);
#4339=VERTEX_POINT('',#15784);
#4340=VERTEX_POINT('',#15817);
#4341=VERTEX_POINT('',#15843);
#4342=VERTEX_POINT('',#15849);
#4343=VERTEX_POINT('',#15855);
#4344=VERTEX_POINT('',#15864);
#4345=VERTEX_POINT('',#15865);
#4346=VERTEX_POINT('',#15870);
#4347=VERTEX_POINT('',#15899);
#4348=VERTEX_POINT('',#15901);
#4349=VERTEX_POINT('',#15930);
#4350=VERTEX_POINT('',#15939);
#4351=VERTEX_POINT('',#15943);
#4352=VERTEX_POINT('',#15950);
#4353=VERTEX_POINT('',#15957);
#4354=VERTEX_POINT('',#15986);
#4355=VERTEX_POINT('',#16052);
#4356=VERTEX_POINT('',#16101);
#4357=VERTEX_POINT('',#16108);
#4358=VERTEX_POINT('',#16146);
#4359=VERTEX_POINT('',#16156);
#4360=VERTEX_POINT('',#16163);
#4361=VERTEX_POINT('',#16192);
#4362=VERTEX_POINT('',#16194);
#4363=VERTEX_POINT('',#16319);
#4364=VERTEX_POINT('',#16326);
#4365=VERTEX_POINT('',#16428);
#4366=VERTEX_POINT('',#16435);
#4367=VERTEX_POINT('',#16464);
#4368=VERTEX_POINT('',#16466);
#4369=VERTEX_POINT('',#16517);
#4370=VERTEX_POINT('',#16546);
#4371=VERTEX_POINT('',#16553);
#4372=VERTEX_POINT('',#16575);
#4373=VERTEX_POINT('',#16610);
#4374=VERTEX_POINT('',#16638);
#4375=VERTEX_POINT('',#16733);
#4376=VERTEX_POINT('',#16734);
#4377=VERTEX_POINT('',#16736);
#4378=VERTEX_POINT('',#16740);
#4379=VERTEX_POINT('',#16741);
#4380=VERTEX_POINT('',#16743);
#4381=VERTEX_POINT('',#16747);
#4382=VERTEX_POINT('',#16748);
#4383=VERTEX_POINT('',#16750);
#4384=VERTEX_POINT('',#16785);
#4385=VERTEX_POINT('',#16786);
#4386=VERTEX_POINT('',#16788);
#5407=EDGE_CURVE('',#4239,#4240,#617,.T.);
#5408=EDGE_CURVE('',#4239,#4240,#3691,.T.);
#5409=EDGE_CURVE('',#4241,#4242,#618,.T.);
#5410=EDGE_CURVE('',#4241,#4242,#3692,.T.);
#5411=EDGE_CURVE('',#4243,#4244,#619,.T.);
#5412=EDGE_CURVE('',#4243,#4244,#3693,.T.);
#5413=EDGE_CURVE('',#4245,#4246,#620,.T.);
#5414=EDGE_CURVE('',#4245,#4246,#3694,.T.);
#5415=EDGE_CURVE('',#4247,#4242,#621,.T.);
#5416=EDGE_CURVE('',#4247,#4248,#622,.T.);
#5417=EDGE_CURVE('',#4249,#4248,#623,.T.);
#5418=EDGE_CURVE('',#4249,#4250,#624,.T.);
#5419=EDGE_CURVE('',#4241,#4250,#625,.T.);
#5420=EDGE_CURVE('',#4251,#4246,#626,.T.);
#5421=EDGE_CURVE('',#4251,#4252,#627,.T.);
#5422=EDGE_CURVE('',#4253,#4252,#628,.T.);
#5423=EDGE_CURVE('',#4253,#4254,#629,.T.);
#5424=EDGE_CURVE('',#4245,#4254,#630,.T.);
#5425=EDGE_CURVE('',#4239,#4255,#631,.T.);
#5426=EDGE_CURVE('',#4255,#4251,#2739,.T.);
#5427=EDGE_CURVE('',#4254,#4256,#2740,.T.);
#5428=EDGE_CURVE('',#4256,#4240,#632,.T.);
#5429=EDGE_CURVE('',#4257,#4257,#3695,.T.);
#5430=EDGE_CURVE('',#4258,#4258,#3696,.T.);
#5431=EDGE_CURVE('',#4259,#4259,#3697,.T.);
#5432=EDGE_CURVE('',#4260,#4260,#3698,.T.);
#5433=EDGE_CURVE('',#4260,#4257,#2741,.T.);
#5434=EDGE_CURVE('',#4261,#4261,#3699,.T.);
#5435=EDGE_CURVE('',#4261,#4262,#2742,.T.);
#5436=EDGE_CURVE('',#4262,#4262,#3700,.T.);
#5437=EDGE_CURVE('',#4263,#4263,#3701,.T.);
#5438=EDGE_CURVE('',#4263,#4264,#2743,.T.);
#5439=EDGE_CURVE('',#4264,#4264,#3702,.T.);
#5440=EDGE_CURVE('',#4265,#4265,#3703,.T.);
#5441=EDGE_CURVE('',#4265,#4258,#2744,.T.);
#5442=EDGE_CURVE('',#4266,#4266,#3704,.T.);
#5443=EDGE_CURVE('',#4266,#4267,#2745,.T.);
#5444=EDGE_CURVE('',#4267,#4267,#3705,.T.);
#5445=EDGE_CURVE('',#4268,#4268,#3706,.T.);
#5446=EDGE_CURVE('',#4269,#4269,#3707,.T.);
#5447=EDGE_CURVE('',#4269,#4270,#2746,.T.);
#5448=EDGE_CURVE('',#4270,#4270,#3708,.T.);
#5449=EDGE_CURVE('',#4271,#4271,#3709,.T.);
#5450=EDGE_CURVE('',#4268,#4272,#2747,.T.);
#5451=EDGE_CURVE('',#4272,#4272,#3710,.T.);
#5452=EDGE_CURVE('',#4271,#4273,#2748,.T.);
#5453=EDGE_CURVE('',#4273,#4273,#3711,.T.);
#5454=EDGE_CURVE('',#4274,#4275,#2749,.T.);
#5455=EDGE_CURVE('',#4276,#4274,#2750,.T.);
#5456=EDGE_CURVE('',#4277,#4276,#2751,.T.);
#5457=EDGE_CURVE('',#4277,#4275,#2752,.T.);
#5458=EDGE_CURVE('',#4278,#4279,#2753,.T.);
#5459=EDGE_CURVE('',#4278,#4280,#2754,.T.);
#5460=EDGE_CURVE('',#4281,#4280,#2755,.T.);
#5461=EDGE_CURVE('',#4279,#4281,#2756,.T.);
#5462=EDGE_CURVE('',#4282,#4283,#2757,.T.);
#5463=EDGE_CURVE('',#4282,#4284,#2758,.T.);
#5464=EDGE_CURVE('',#4285,#4284,#2759,.T.);
#5465=EDGE_CURVE('',#4283,#4285,#2760,.T.);
#5466=EDGE_CURVE('',#4286,#4287,#2761,.T.);
#5467=EDGE_CURVE('',#4286,#4288,#2762,.T.);
#5468=EDGE_CURVE('',#4289,#4288,#2763,.T.);
#5469=EDGE_CURVE('',#4287,#4289,#2764,.T.);
#5470=EDGE_CURVE('',#4290,#4291,#2765,.T.);
#5471=EDGE_CURVE('',#4290,#4292,#2766,.T.);
#5472=EDGE_CURVE('',#4293,#4292,#2767,.T.);
#5473=EDGE_CURVE('',#4291,#4293,#2768,.T.);
#5474=EDGE_CURVE('',#4294,#4295,#2769,.T.);
#5475=EDGE_CURVE('',#4296,#4294,#2770,.T.);
#5476=EDGE_CURVE('',#4297,#4296,#2771,.T.);
#5477=EDGE_CURVE('',#4297,#4295,#2772,.T.);
#5478=EDGE_CURVE('',#4298,#4299,#2773,.T.);
#5479=EDGE_CURVE('',#4300,#4298,#2774,.T.);
#5480=EDGE_CURVE('',#4301,#4300,#2775,.T.);
#5481=EDGE_CURVE('',#4301,#4299,#2776,.T.);
#5482=EDGE_CURVE('',#4302,#4302,#3712,.T.);
#5483=EDGE_CURVE('',#4303,#4303,#3713,.T.);
#5484=EDGE_CURVE('',#4275,#4290,#2777,.T.);
#5485=EDGE_CURVE('',#4292,#4277,#2778,.T.);
#5486=EDGE_CURVE('',#4295,#4278,#2779,.T.);
#5487=EDGE_CURVE('',#4280,#4297,#2780,.T.);
#5488=EDGE_CURVE('',#4299,#4282,#2781,.T.);
#5489=EDGE_CURVE('',#4284,#4301,#2782,.T.);
#5490=EDGE_CURVE('',#4304,#4286,#2783,.T.);
#5491=EDGE_CURVE('',#4305,#4304,#2784,.T.);
#5492=EDGE_CURVE('',#4288,#4305,#2785,.T.);
#5493=EDGE_CURVE('',#4306,#4304,#2786,.T.);
#5494=EDGE_CURVE('',#4307,#4306,#2787,.T.);
#5495=EDGE_CURVE('',#4305,#4307,#2788,.T.);
#5496=EDGE_CURVE('',#4308,#4309,#2789,.T.);
#5497=EDGE_CURVE('',#4310,#4309,#633,.T.);
#5498=EDGE_CURVE('',#4256,#4310,#634,.T.);
#5499=EDGE_CURVE('',#4308,#4253,#635,.T.);
#5500=EDGE_CURVE('',#4307,#4311,#2790,.T.);
#5501=EDGE_CURVE('',#4252,#4311,#636,.T.);
#5502=EDGE_CURVE('',#4312,#4255,#637,.T.);
#5503=EDGE_CURVE('',#4313,#4312,#638,.T.);
#5504=EDGE_CURVE('',#4313,#4289,#2791,.T.);
#5505=EDGE_CURVE('',#4300,#4314,#2792,.T.);
#5506=EDGE_CURVE('',#4315,#4314,#639,.T.);
#5507=EDGE_CURVE('',#4316,#4315,#640,.T.);
#5508=EDGE_CURVE('',#4317,#4316,#2793,.T.);
#5509=EDGE_CURVE('',#4318,#4317,#641,.T.);
#5510=EDGE_CURVE('',#4319,#4318,#642,.T.);
#5511=EDGE_CURVE('',#4319,#4285,#2794,.T.);
#5512=EDGE_CURVE('',#4296,#4320,#2795,.T.);
#5513=EDGE_CURVE('',#4248,#4320,#643,.T.);
#5514=EDGE_CURVE('',#4321,#4247,#2796,.T.);
#5515=EDGE_CURVE('',#4322,#4321,#644,.T.);
#5516=EDGE_CURVE('',#4323,#4322,#645,.T.);
#5517=EDGE_CURVE('',#4323,#4281,#2797,.T.);
#5518=EDGE_CURVE('',#4324,#4291,#2798,.T.);
#5519=EDGE_CURVE('',#4324,#4325,#646,.T.);
#5520=EDGE_CURVE('',#4325,#4326,#2799,.T.);
#5521=EDGE_CURVE('',#4326,#4327,#647,.T.);
#5522=EDGE_CURVE('',#4274,#4327,#2800,.T.);
#5523=EDGE_CURVE('',#4313,#4309,#648,.T.);
#5524=EDGE_CURVE('',#4308,#4311,#649,.T.);
#5525=EDGE_CURVE('',#4328,#4306,#2801,.T.);
#5526=EDGE_CURVE('',#4328,#4314,#650,.T.);
#5527=EDGE_CURVE('',#4329,#4298,#2802,.T.);
#5528=EDGE_CURVE('',#4329,#4320,#651,.T.);
#5529=EDGE_CURVE('',#4330,#4294,#2803,.T.);
#5530=EDGE_CURVE('',#4330,#4331,#652,.T.);
#5531=EDGE_CURVE('',#4331,#4324,#653,.T.);
#5532=EDGE_CURVE('',#4293,#4332,#2804,.T.);
#5533=EDGE_CURVE('',#4333,#4332,#654,.T.);
#5534=EDGE_CURVE('',#4333,#4334,#655,.T.);
#5535=EDGE_CURVE('',#4335,#4334,#656,.T.);
#5536=EDGE_CURVE('',#4335,#4336,#2805,.T.);
#5537=EDGE_CURVE('',#4337,#4336,#657,.T.);
#5538=EDGE_CURVE('',#4337,#4338,#658,.T.);
#5539=EDGE_CURVE('',#4339,#4338,#659,.T.);
#5540=EDGE_CURVE('',#4339,#4276,#2806,.T.);
#5541=EDGE_CURVE('',#4327,#4340,#660,.T.);
#5542=EDGE_CURVE('',#4340,#4341,#661,.T.);
#5543=EDGE_CURVE('',#4279,#4341,#2807,.T.);
#5544=EDGE_CURVE('',#4323,#4342,#662,.T.);
#5545=EDGE_CURVE('',#4283,#4342,#2808,.T.);
#5546=EDGE_CURVE('',#4319,#4343,#663,.T.);
#5547=EDGE_CURVE('',#4287,#4343,#2809,.T.);
#5548=EDGE_CURVE('',#4344,#4345,#664,.T.);
#5549=EDGE_CURVE('',#4345,#4346,#665,.T.);
#5550=EDGE_CURVE('',#4346,#4347,#2810,.T.);
#5551=EDGE_CURVE('',#4347,#4348,#666,.T.);
#5552=EDGE_CURVE('',#4348,#4349,#667,.T.);
#5553=EDGE_CURVE('',#4344,#4349,#2811,.T.);
#5554=EDGE_CURVE('',#4259,#4303,#2812,.T.);
#5555=EDGE_CURVE('',#4350,#4350,#3714,.T.);
#5556=EDGE_CURVE('',#4350,#4302,#2813,.T.);
#5557=EDGE_CURVE('',#4344,#4351,#668,.T.);
#5558=EDGE_CURVE('',#4352,#4349,#669,.T.);
#5559=EDGE_CURVE('',#4353,#4352,#670,.T.);
#5560=EDGE_CURVE('',#4354,#4353,#2814,.T.);
#5561=EDGE_CURVE('',#4351,#4354,#671,.T.);
#5562=EDGE_CURVE('',#4312,#4310,#672,.T.);
#5563=EDGE_CURVE('',#4351,#4355,#673,.T.);
#5564=EDGE_CURVE('',#4355,#4345,#674,.T.);
#5565=EDGE_CURVE('',#4356,#4354,#675,.T.);
#5566=EDGE_CURVE('',#4355,#4356,#3715,.F.);
#5567=EDGE_CURVE('',#4353,#4357,#676,.T.);
#5568=EDGE_CURVE('',#4357,#4356,#2815,.T.);
#5569=EDGE_CURVE('',#4348,#4358,#677,.T.);
#5570=EDGE_CURVE('',#4358,#4352,#678,.T.);
#5571=EDGE_CURVE('',#4359,#4343,#679,.T.);
#5572=EDGE_CURVE('',#4360,#4359,#680,.T.);
#5573=EDGE_CURVE('',#4361,#4360,#2816,.T.);
#5574=EDGE_CURVE('',#4362,#4361,#681,.T.);
#5575=EDGE_CURVE('',#4328,#4362,#682,.T.);
#5576=EDGE_CURVE('',#4318,#4359,#683,.T.);
#5577=EDGE_CURVE('',#4360,#4317,#684,.T.);
#5578=EDGE_CURVE('',#4316,#4361,#685,.T.);
#5579=EDGE_CURVE('',#4362,#4315,#686,.T.);
#5580=EDGE_CURVE('',#4363,#4342,#687,.T.);
#5581=EDGE_CURVE('',#4364,#4363,#688,.T.);
#5582=EDGE_CURVE('',#4250,#4364,#2817,.T.);
#5583=EDGE_CURVE('',#4329,#4249,#689,.T.);
#5584=EDGE_CURVE('',#4322,#4363,#690,.T.);
#5585=EDGE_CURVE('',#4364,#4244,#691,.T.);
#5586=EDGE_CURVE('',#4243,#4321,#692,.T.);
#5587=EDGE_CURVE('',#4365,#4341,#693,.T.);
#5588=EDGE_CURVE('',#4366,#4365,#694,.T.);
#5589=EDGE_CURVE('',#4367,#4366,#2818,.T.);
#5590=EDGE_CURVE('',#4368,#4367,#695,.T.);
#5591=EDGE_CURVE('',#4330,#4368,#696,.T.);
#5592=EDGE_CURVE('',#4340,#4369,#697,.T.);
#5593=EDGE_CURVE('',#4369,#4365,#698,.T.);
#5594=EDGE_CURVE('',#4370,#4369,#3716,.F.);
#5595=EDGE_CURVE('',#4366,#4370,#699,.T.);
#5596=EDGE_CURVE('',#4370,#4371,#2819,.T.);
#5597=EDGE_CURVE('',#4371,#4367,#700,.T.);
#5598=EDGE_CURVE('',#4368,#4372,#701,.T.);
#5599=EDGE_CURVE('',#4372,#4331,#702,.T.);
#5600=EDGE_CURVE('',#4372,#4371,#3717,.F.);
#5601=EDGE_CURVE('',#4371,#4325,#3718,.F.);
#5602=EDGE_CURVE('',#4325,#4372,#3719,.F.);
#5603=EDGE_CURVE('',#4357,#4358,#3720,.F.);
#5604=EDGE_CURVE('',#4358,#4373,#3721,.F.);
#5605=EDGE_CURVE('',#4373,#4357,#3722,.F.);
#5606=EDGE_CURVE('',#4369,#4326,#3723,.F.);
#5607=EDGE_CURVE('',#4326,#4370,#3724,.F.);
#5608=EDGE_CURVE('',#4374,#4355,#3725,.F.);
#5609=EDGE_CURVE('',#4356,#4374,#3726,.F.);
#5610=EDGE_CURVE('',#4374,#4373,#2820,.T.);
#5611=EDGE_CURVE('',#4346,#4374,#703,.T.);
#5612=EDGE_CURVE('',#4373,#4347,#704,.T.);
#5613=EDGE_CURVE('',#4375,#4376,#3727,.F.);
#5614=EDGE_CURVE('',#4377,#4375,#3728,.F.);
#5615=EDGE_CURVE('',#4376,#4377,#3729,.F.);
#5616=EDGE_CURVE('',#4378,#4379,#3730,.F.);
#5617=EDGE_CURVE('',#4380,#4378,#3731,.F.);
#5618=EDGE_CURVE('',#4379,#4380,#3732,.F.);
#5619=EDGE_CURVE('',#4381,#4382,#3733,.F.);
#5620=EDGE_CURVE('',#4383,#4381,#3734,.F.);
#5621=EDGE_CURVE('',#4382,#4383,#3735,.F.);
#5622=EDGE_CURVE('',#4376,#4383,#2821,.T.);
#5623=EDGE_CURVE('',#4381,#4375,#2822,.T.);
#5624=EDGE_CURVE('',#4338,#4382,#705,.T.);
#5625=EDGE_CURVE('',#4383,#4339,#706,.T.);
#5626=EDGE_CURVE('',#4384,#4385,#3736,.F.);
#5627=EDGE_CURVE('',#4386,#4384,#3737,.F.);
#5628=EDGE_CURVE('',#4385,#4386,#3738,.F.);
#5629=EDGE_CURVE('',#4384,#4380,#2823,.T.);
#5630=EDGE_CURVE('',#4378,#4386,#2824,.T.);
#5631=EDGE_CURVE('',#4382,#4385,#707,.T.);
#5632=EDGE_CURVE('',#4386,#4381,#708,.T.);
#5633=EDGE_CURVE('',#4336,#4384,#709,.T.);
#5634=EDGE_CURVE('',#4385,#4337,#710,.T.);
#5635=EDGE_CURVE('',#4334,#4379,#711,.T.);
#5636=EDGE_CURVE('',#4380,#4335,#712,.T.);
#5637=EDGE_CURVE('',#4379,#4377,#713,.T.);
#5638=EDGE_CURVE('',#4375,#4378,#714,.T.);
#5639=EDGE_CURVE('',#4332,#4376,#715,.T.);
#5640=EDGE_CURVE('',#4377,#4333,#716,.T.);
#7497=ORIENTED_EDGE('',*,*,#5407,.F.);
#7498=ORIENTED_EDGE('',*,*,#5408,.T.);
#7499=ORIENTED_EDGE('',*,*,#5409,.F.);
#7500=ORIENTED_EDGE('',*,*,#5410,.T.);
#7501=ORIENTED_EDGE('',*,*,#5411,.F.);
#7502=ORIENTED_EDGE('',*,*,#5412,.T.);
#7503=ORIENTED_EDGE('',*,*,#5413,.F.);
#7504=ORIENTED_EDGE('',*,*,#5414,.T.);
#7505=ORIENTED_EDGE('',*,*,#5409,.T.);
#7506=ORIENTED_EDGE('',*,*,#5415,.F.);
#7507=ORIENTED_EDGE('',*,*,#5416,.T.);
#7508=ORIENTED_EDGE('',*,*,#5417,.F.);
#7509=ORIENTED_EDGE('',*,*,#5418,.T.);
#7510=ORIENTED_EDGE('',*,*,#5419,.F.);
#7511=ORIENTED_EDGE('',*,*,#5413,.T.);
#7512=ORIENTED_EDGE('',*,*,#5420,.F.);
#7513=ORIENTED_EDGE('',*,*,#5421,.T.);
#7514=ORIENTED_EDGE('',*,*,#5422,.F.);
#7515=ORIENTED_EDGE('',*,*,#5423,.T.);
#7516=ORIENTED_EDGE('',*,*,#5424,.F.);
#7517=ORIENTED_EDGE('',*,*,#5425,.T.);
#7518=ORIENTED_EDGE('',*,*,#5426,.T.);
#7519=ORIENTED_EDGE('',*,*,#5420,.T.);
#7520=ORIENTED_EDGE('',*,*,#5414,.F.);
#7521=ORIENTED_EDGE('',*,*,#5424,.T.);
#7522=ORIENTED_EDGE('',*,*,#5427,.T.);
#7523=ORIENTED_EDGE('',*,*,#5428,.T.);
#7524=ORIENTED_EDGE('',*,*,#5408,.F.);
#7525=ORIENTED_EDGE('',*,*,#5429,.T.);
#7526=ORIENTED_EDGE('',*,*,#5430,.T.);
#7527=ORIENTED_EDGE('',*,*,#5431,.T.);
#7528=ORIENTED_EDGE('',*,*,#5432,.F.);
#7529=ORIENTED_EDGE('',*,*,#5433,.T.);
#7530=ORIENTED_EDGE('',*,*,#5429,.F.);
#7531=ORIENTED_EDGE('',*,*,#5433,.F.);
#7532=ORIENTED_EDGE('',*,*,#5434,.F.);
#7533=ORIENTED_EDGE('',*,*,#5435,.T.);
#7534=ORIENTED_EDGE('',*,*,#5436,.F.);
#7535=ORIENTED_EDGE('',*,*,#5435,.F.);
#7536=ORIENTED_EDGE('',*,*,#5437,.F.);
#7537=ORIENTED_EDGE('',*,*,#5438,.T.);
#7538=ORIENTED_EDGE('',*,*,#5439,.F.);
#7539=ORIENTED_EDGE('',*,*,#5438,.F.);
#7540=ORIENTED_EDGE('',*,*,#5440,.F.);
#7541=ORIENTED_EDGE('',*,*,#5441,.T.);
#7542=ORIENTED_EDGE('',*,*,#5430,.F.);
#7543=ORIENTED_EDGE('',*,*,#5441,.F.);
#7544=ORIENTED_EDGE('',*,*,#5442,.F.);
#7545=ORIENTED_EDGE('',*,*,#5443,.T.);
#7546=ORIENTED_EDGE('',*,*,#5444,.T.);
#7547=ORIENTED_EDGE('',*,*,#5443,.F.);
#7548=ORIENTED_EDGE('',*,*,#5444,.F.);
#7549=ORIENTED_EDGE('',*,*,#5445,.F.);
#7550=ORIENTED_EDGE('',*,*,#5446,.F.);
#7551=ORIENTED_EDGE('',*,*,#5447,.T.);
#7552=ORIENTED_EDGE('',*,*,#5448,.T.);
#7553=ORIENTED_EDGE('',*,*,#5447,.F.);
#7554=ORIENTED_EDGE('',*,*,#5448,.F.);
#7555=ORIENTED_EDGE('',*,*,#5449,.F.);
#7556=ORIENTED_EDGE('',*,*,#5445,.T.);
#7557=ORIENTED_EDGE('',*,*,#5450,.T.);
#7558=ORIENTED_EDGE('',*,*,#5451,.F.);
#7559=ORIENTED_EDGE('',*,*,#5450,.F.);
#7560=ORIENTED_EDGE('',*,*,#5449,.T.);
#7561=ORIENTED_EDGE('',*,*,#5452,.T.);
#7562=ORIENTED_EDGE('',*,*,#5453,.F.);
#7563=ORIENTED_EDGE('',*,*,#5452,.F.);
#7564=ORIENTED_EDGE('',*,*,#5454,.F.);
#7565=ORIENTED_EDGE('',*,*,#5455,.F.);
#7566=ORIENTED_EDGE('',*,*,#5456,.F.);
#7567=ORIENTED_EDGE('',*,*,#5457,.T.);
#7568=ORIENTED_EDGE('',*,*,#5458,.F.);
#7569=ORIENTED_EDGE('',*,*,#5459,.T.);
#7570=ORIENTED_EDGE('',*,*,#5460,.F.);
#7571=ORIENTED_EDGE('',*,*,#5461,.F.);
#7572=ORIENTED_EDGE('',*,*,#5462,.F.);
#7573=ORIENTED_EDGE('',*,*,#5463,.T.);
#7574=ORIENTED_EDGE('',*,*,#5464,.F.);
#7575=ORIENTED_EDGE('',*,*,#5465,.F.);
#7576=ORIENTED_EDGE('',*,*,#5466,.F.);
#7577=ORIENTED_EDGE('',*,*,#5467,.T.);
#7578=ORIENTED_EDGE('',*,*,#5468,.F.);
#7579=ORIENTED_EDGE('',*,*,#5469,.F.);
#7580=ORIENTED_EDGE('',*,*,#5470,.F.);
#7581=ORIENTED_EDGE('',*,*,#5471,.T.);
#7582=ORIENTED_EDGE('',*,*,#5472,.F.);
#7583=ORIENTED_EDGE('',*,*,#5473,.F.);
#7584=ORIENTED_EDGE('',*,*,#5474,.F.);
#7585=ORIENTED_EDGE('',*,*,#5475,.F.);
#7586=ORIENTED_EDGE('',*,*,#5476,.F.);
#7587=ORIENTED_EDGE('',*,*,#5477,.T.);
#7588=ORIENTED_EDGE('',*,*,#5478,.F.);
#7589=ORIENTED_EDGE('',*,*,#5479,.F.);
#7590=ORIENTED_EDGE('',*,*,#5480,.F.);
#7591=ORIENTED_EDGE('',*,*,#5481,.T.);
#7592=ORIENTED_EDGE('',*,*,#5482,.F.);
#7593=ORIENTED_EDGE('',*,*,#5451,.T.);
#7594=ORIENTED_EDGE('',*,*,#5483,.F.);
#7595=ORIENTED_EDGE('',*,*,#5453,.T.);
#7596=ORIENTED_EDGE('',*,*,#5484,.F.);
#7597=ORIENTED_EDGE('',*,*,#5457,.F.);
#7598=ORIENTED_EDGE('',*,*,#5485,.F.);
#7599=ORIENTED_EDGE('',*,*,#5471,.F.);
#7600=ORIENTED_EDGE('',*,*,#5486,.F.);
#7601=ORIENTED_EDGE('',*,*,#5477,.F.);
#7602=ORIENTED_EDGE('',*,*,#5487,.F.);
#7603=ORIENTED_EDGE('',*,*,#5459,.F.);
#7604=ORIENTED_EDGE('',*,*,#5488,.F.);
#7605=ORIENTED_EDGE('',*,*,#5481,.F.);
#7606=ORIENTED_EDGE('',*,*,#5489,.F.);
#7607=ORIENTED_EDGE('',*,*,#5463,.F.);
#7608=ORIENTED_EDGE('',*,*,#5490,.F.);
#7609=ORIENTED_EDGE('',*,*,#5491,.F.);
#7610=ORIENTED_EDGE('',*,*,#5492,.F.);
#7611=ORIENTED_EDGE('',*,*,#5467,.F.);
#7612=ORIENTED_EDGE('',*,*,#5493,.F.);
#7613=ORIENTED_EDGE('',*,*,#5494,.F.);
#7614=ORIENTED_EDGE('',*,*,#5495,.F.);
#7615=ORIENTED_EDGE('',*,*,#5491,.T.);
#7616=ORIENTED_EDGE('',*,*,#5496,.T.);
#7617=ORIENTED_EDGE('',*,*,#5497,.F.);
#7618=ORIENTED_EDGE('',*,*,#5498,.F.);
#7619=ORIENTED_EDGE('',*,*,#5427,.F.);
#7620=ORIENTED_EDGE('',*,*,#5423,.F.);
#7621=ORIENTED_EDGE('',*,*,#5499,.F.);
#7622=ORIENTED_EDGE('',*,*,#5468,.T.);
#7623=ORIENTED_EDGE('',*,*,#5492,.T.);
#7624=ORIENTED_EDGE('',*,*,#5495,.T.);
#7625=ORIENTED_EDGE('',*,*,#5500,.T.);
#7626=ORIENTED_EDGE('',*,*,#5501,.F.);
#7627=ORIENTED_EDGE('',*,*,#5421,.F.);
#7628=ORIENTED_EDGE('',*,*,#5426,.F.);
#7629=ORIENTED_EDGE('',*,*,#5502,.F.);
#7630=ORIENTED_EDGE('',*,*,#5503,.F.);
#7631=ORIENTED_EDGE('',*,*,#5504,.T.);
#7632=ORIENTED_EDGE('',*,*,#5464,.T.);
#7633=ORIENTED_EDGE('',*,*,#5489,.T.);
#7634=ORIENTED_EDGE('',*,*,#5480,.T.);
#7635=ORIENTED_EDGE('',*,*,#5505,.T.);
#7636=ORIENTED_EDGE('',*,*,#5506,.F.);
#7637=ORIENTED_EDGE('',*,*,#5507,.F.);
#7638=ORIENTED_EDGE('',*,*,#5508,.F.);
#7639=ORIENTED_EDGE('',*,*,#5509,.F.);
#7640=ORIENTED_EDGE('',*,*,#5510,.F.);
#7641=ORIENTED_EDGE('',*,*,#5511,.T.);
#7642=ORIENTED_EDGE('',*,*,#5460,.T.);
#7643=ORIENTED_EDGE('',*,*,#5487,.T.);
#7644=ORIENTED_EDGE('',*,*,#5476,.T.);
#7645=ORIENTED_EDGE('',*,*,#5512,.T.);
#7646=ORIENTED_EDGE('',*,*,#5513,.F.);
#7647=ORIENTED_EDGE('',*,*,#5416,.F.);
#7648=ORIENTED_EDGE('',*,*,#5514,.F.);
#7649=ORIENTED_EDGE('',*,*,#5515,.F.);
#7650=ORIENTED_EDGE('',*,*,#5516,.F.);
#7651=ORIENTED_EDGE('',*,*,#5517,.T.);
#7652=ORIENTED_EDGE('',*,*,#5454,.T.);
#7653=ORIENTED_EDGE('',*,*,#5484,.T.);
#7654=ORIENTED_EDGE('',*,*,#5470,.T.);
#7655=ORIENTED_EDGE('',*,*,#5518,.F.);
#7656=ORIENTED_EDGE('',*,*,#5519,.T.);
#7657=ORIENTED_EDGE('',*,*,#5520,.T.);
#7658=ORIENTED_EDGE('',*,*,#5521,.T.);
#7659=ORIENTED_EDGE('',*,*,#5522,.F.);
#7660=ORIENTED_EDGE('',*,*,#5469,.T.);
#7661=ORIENTED_EDGE('',*,*,#5504,.F.);
#7662=ORIENTED_EDGE('',*,*,#5523,.T.);
#7663=ORIENTED_EDGE('',*,*,#5496,.F.);
#7664=ORIENTED_EDGE('',*,*,#5524,.T.);
#7665=ORIENTED_EDGE('',*,*,#5500,.F.);
#7666=ORIENTED_EDGE('',*,*,#5494,.T.);
#7667=ORIENTED_EDGE('',*,*,#5525,.F.);
#7668=ORIENTED_EDGE('',*,*,#5526,.T.);
#7669=ORIENTED_EDGE('',*,*,#5505,.F.);
#7670=ORIENTED_EDGE('',*,*,#5479,.T.);
#7671=ORIENTED_EDGE('',*,*,#5527,.F.);
#7672=ORIENTED_EDGE('',*,*,#5528,.T.);
#7673=ORIENTED_EDGE('',*,*,#5512,.F.);
#7674=ORIENTED_EDGE('',*,*,#5475,.T.);
#7675=ORIENTED_EDGE('',*,*,#5529,.F.);
#7676=ORIENTED_EDGE('',*,*,#5530,.T.);
#7677=ORIENTED_EDGE('',*,*,#5531,.T.);
#7678=ORIENTED_EDGE('',*,*,#5518,.T.);
#7679=ORIENTED_EDGE('',*,*,#5473,.T.);
#7680=ORIENTED_EDGE('',*,*,#5532,.T.);
#7681=ORIENTED_EDGE('',*,*,#5533,.F.);
#7682=ORIENTED_EDGE('',*,*,#5534,.T.);
#7683=ORIENTED_EDGE('',*,*,#5535,.F.);
#7684=ORIENTED_EDGE('',*,*,#5536,.T.);
#7685=ORIENTED_EDGE('',*,*,#5537,.F.);
#7686=ORIENTED_EDGE('',*,*,#5538,.T.);
#7687=ORIENTED_EDGE('',*,*,#5539,.F.);
#7688=ORIENTED_EDGE('',*,*,#5540,.T.);
#7689=ORIENTED_EDGE('',*,*,#5455,.T.);
#7690=ORIENTED_EDGE('',*,*,#5522,.T.);
#7691=ORIENTED_EDGE('',*,*,#5541,.T.);
#7692=ORIENTED_EDGE('',*,*,#5542,.T.);
#7693=ORIENTED_EDGE('',*,*,#5543,.F.);
#7694=ORIENTED_EDGE('',*,*,#5461,.T.);
#7695=ORIENTED_EDGE('',*,*,#5517,.F.);
#7696=ORIENTED_EDGE('',*,*,#5544,.T.);
#7697=ORIENTED_EDGE('',*,*,#5545,.F.);
#7698=ORIENTED_EDGE('',*,*,#5465,.T.);
#7699=ORIENTED_EDGE('',*,*,#5511,.F.);
#7700=ORIENTED_EDGE('',*,*,#5546,.T.);
#7701=ORIENTED_EDGE('',*,*,#5547,.F.);
#7702=ORIENTED_EDGE('',*,*,#5548,.T.);
#7703=ORIENTED_EDGE('',*,*,#5549,.T.);
#7704=ORIENTED_EDGE('',*,*,#5550,.T.);
#7705=ORIENTED_EDGE('',*,*,#5551,.T.);
#7706=ORIENTED_EDGE('',*,*,#5552,.T.);
#7707=ORIENTED_EDGE('',*,*,#5553,.F.);
#7708=ORIENTED_EDGE('',*,*,#5431,.F.);
#7709=ORIENTED_EDGE('',*,*,#5554,.T.);
#7710=ORIENTED_EDGE('',*,*,#5483,.T.);
#7711=ORIENTED_EDGE('',*,*,#5554,.F.);
#7712=ORIENTED_EDGE('',*,*,#5555,.F.);
#7713=ORIENTED_EDGE('',*,*,#5556,.T.);
#7714=ORIENTED_EDGE('',*,*,#5482,.T.);
#7715=ORIENTED_EDGE('',*,*,#5556,.F.);
#7716=ORIENTED_EDGE('',*,*,#5557,.F.);
#7717=ORIENTED_EDGE('',*,*,#5553,.T.);
#7718=ORIENTED_EDGE('',*,*,#5558,.F.);
#7719=ORIENTED_EDGE('',*,*,#5559,.F.);
#7720=ORIENTED_EDGE('',*,*,#5560,.F.);
#7721=ORIENTED_EDGE('',*,*,#5561,.F.);
#7722=ORIENTED_EDGE('',*,*,#5497,.T.);
#7723=ORIENTED_EDGE('',*,*,#5523,.F.);
#7724=ORIENTED_EDGE('',*,*,#5503,.T.);
#7725=ORIENTED_EDGE('',*,*,#5562,.T.);
#7726=ORIENTED_EDGE('',*,*,#5557,.T.);
#7727=ORIENTED_EDGE('',*,*,#5563,.T.);
#7728=ORIENTED_EDGE('',*,*,#5564,.T.);
#7729=ORIENTED_EDGE('',*,*,#5548,.F.);
#7730=ORIENTED_EDGE('',*,*,#5407,.T.);
#7731=ORIENTED_EDGE('',*,*,#5428,.F.);
#7732=ORIENTED_EDGE('',*,*,#5498,.T.);
#7733=ORIENTED_EDGE('',*,*,#5562,.F.);
#7734=ORIENTED_EDGE('',*,*,#5502,.T.);
#7735=ORIENTED_EDGE('',*,*,#5425,.F.);
#7736=ORIENTED_EDGE('',*,*,#5561,.T.);
#7737=ORIENTED_EDGE('',*,*,#5565,.F.);
#7738=ORIENTED_EDGE('',*,*,#5566,.F.);
#7739=ORIENTED_EDGE('',*,*,#5563,.F.);
#7740=ORIENTED_EDGE('',*,*,#5560,.T.);
#7741=ORIENTED_EDGE('',*,*,#5567,.T.);
#7742=ORIENTED_EDGE('',*,*,#5568,.T.);
#7743=ORIENTED_EDGE('',*,*,#5565,.T.);
#7744=ORIENTED_EDGE('',*,*,#5499,.T.);
#7745=ORIENTED_EDGE('',*,*,#5422,.T.);
#7746=ORIENTED_EDGE('',*,*,#5501,.T.);
#7747=ORIENTED_EDGE('',*,*,#5524,.F.);
#7748=ORIENTED_EDGE('',*,*,#5558,.T.);
#7749=ORIENTED_EDGE('',*,*,#5552,.F.);
#7750=ORIENTED_EDGE('',*,*,#5569,.T.);
#7751=ORIENTED_EDGE('',*,*,#5570,.T.);
#7752=ORIENTED_EDGE('',*,*,#5466,.T.);
#7753=ORIENTED_EDGE('',*,*,#5547,.T.);
#7754=ORIENTED_EDGE('',*,*,#5571,.F.);
#7755=ORIENTED_EDGE('',*,*,#5572,.F.);
#7756=ORIENTED_EDGE('',*,*,#5573,.F.);
#7757=ORIENTED_EDGE('',*,*,#5574,.F.);
#7758=ORIENTED_EDGE('',*,*,#5575,.F.);
#7759=ORIENTED_EDGE('',*,*,#5525,.T.);
#7760=ORIENTED_EDGE('',*,*,#5493,.T.);
#7761=ORIENTED_EDGE('',*,*,#5490,.T.);
#7762=ORIENTED_EDGE('',*,*,#5571,.T.);
#7763=ORIENTED_EDGE('',*,*,#5546,.F.);
#7764=ORIENTED_EDGE('',*,*,#5510,.T.);
#7765=ORIENTED_EDGE('',*,*,#5576,.T.);
#7766=ORIENTED_EDGE('',*,*,#5572,.T.);
#7767=ORIENTED_EDGE('',*,*,#5576,.F.);
#7768=ORIENTED_EDGE('',*,*,#5509,.T.);
#7769=ORIENTED_EDGE('',*,*,#5577,.F.);
#7770=ORIENTED_EDGE('',*,*,#5573,.T.);
#7771=ORIENTED_EDGE('',*,*,#5577,.T.);
#7772=ORIENTED_EDGE('',*,*,#5508,.T.);
#7773=ORIENTED_EDGE('',*,*,#5578,.T.);
#7774=ORIENTED_EDGE('',*,*,#5574,.T.);
#7775=ORIENTED_EDGE('',*,*,#5578,.F.);
#7776=ORIENTED_EDGE('',*,*,#5507,.T.);
#7777=ORIENTED_EDGE('',*,*,#5579,.F.);
#7778=ORIENTED_EDGE('',*,*,#5575,.T.);
#7779=ORIENTED_EDGE('',*,*,#5579,.T.);
#7780=ORIENTED_EDGE('',*,*,#5506,.T.);
#7781=ORIENTED_EDGE('',*,*,#5526,.F.);
#7782=ORIENTED_EDGE('',*,*,#5462,.T.);
#7783=ORIENTED_EDGE('',*,*,#5545,.T.);
#7784=ORIENTED_EDGE('',*,*,#5580,.F.);
#7785=ORIENTED_EDGE('',*,*,#5581,.F.);
#7786=ORIENTED_EDGE('',*,*,#5582,.F.);
#7787=ORIENTED_EDGE('',*,*,#5418,.F.);
#7788=ORIENTED_EDGE('',*,*,#5583,.F.);
#7789=ORIENTED_EDGE('',*,*,#5527,.T.);
#7790=ORIENTED_EDGE('',*,*,#5478,.T.);
#7791=ORIENTED_EDGE('',*,*,#5488,.T.);
#7792=ORIENTED_EDGE('',*,*,#5580,.T.);
#7793=ORIENTED_EDGE('',*,*,#5544,.F.);
#7794=ORIENTED_EDGE('',*,*,#5516,.T.);
#7795=ORIENTED_EDGE('',*,*,#5584,.T.);
#7796=ORIENTED_EDGE('',*,*,#5411,.T.);
#7797=ORIENTED_EDGE('',*,*,#5585,.F.);
#7798=ORIENTED_EDGE('',*,*,#5581,.T.);
#7799=ORIENTED_EDGE('',*,*,#5584,.F.);
#7800=ORIENTED_EDGE('',*,*,#5515,.T.);
#7801=ORIENTED_EDGE('',*,*,#5586,.F.);
#7802=ORIENTED_EDGE('',*,*,#5419,.T.);
#7803=ORIENTED_EDGE('',*,*,#5582,.T.);
#7804=ORIENTED_EDGE('',*,*,#5585,.T.);
#7805=ORIENTED_EDGE('',*,*,#5412,.F.);
#7806=ORIENTED_EDGE('',*,*,#5586,.T.);
#7807=ORIENTED_EDGE('',*,*,#5514,.T.);
#7808=ORIENTED_EDGE('',*,*,#5415,.T.);
#7809=ORIENTED_EDGE('',*,*,#5410,.F.);
#7810=ORIENTED_EDGE('',*,*,#5439,.T.);
#7811=ORIENTED_EDGE('',*,*,#5436,.T.);
#7812=ORIENTED_EDGE('',*,*,#5555,.T.);
#7813=ORIENTED_EDGE('',*,*,#5583,.T.);
#7814=ORIENTED_EDGE('',*,*,#5417,.T.);
#7815=ORIENTED_EDGE('',*,*,#5513,.T.);
#7816=ORIENTED_EDGE('',*,*,#5528,.F.);
#7817=ORIENTED_EDGE('',*,*,#5458,.T.);
#7818=ORIENTED_EDGE('',*,*,#5543,.T.);
#7819=ORIENTED_EDGE('',*,*,#5587,.F.);
#7820=ORIENTED_EDGE('',*,*,#5588,.F.);
#7821=ORIENTED_EDGE('',*,*,#5589,.F.);
#7822=ORIENTED_EDGE('',*,*,#5590,.F.);
#7823=ORIENTED_EDGE('',*,*,#5591,.F.);
#7824=ORIENTED_EDGE('',*,*,#5529,.T.);
#7825=ORIENTED_EDGE('',*,*,#5474,.T.);
#7826=ORIENTED_EDGE('',*,*,#5486,.T.);
#7827=ORIENTED_EDGE('',*,*,#5587,.T.);
#7828=ORIENTED_EDGE('',*,*,#5542,.F.);
#7829=ORIENTED_EDGE('',*,*,#5592,.T.);
#7830=ORIENTED_EDGE('',*,*,#5593,.T.);
#7831=ORIENTED_EDGE('',*,*,#5588,.T.);
#7832=ORIENTED_EDGE('',*,*,#5593,.F.);
#7833=ORIENTED_EDGE('',*,*,#5594,.F.);
#7834=ORIENTED_EDGE('',*,*,#5595,.F.);
#7835=ORIENTED_EDGE('',*,*,#5589,.T.);
#7836=ORIENTED_EDGE('',*,*,#5595,.T.);
#7837=ORIENTED_EDGE('',*,*,#5596,.T.);
#7838=ORIENTED_EDGE('',*,*,#5597,.T.);
#7839=ORIENTED_EDGE('',*,*,#5591,.T.);
#7840=ORIENTED_EDGE('',*,*,#5598,.T.);
#7841=ORIENTED_EDGE('',*,*,#5599,.T.);
#7842=ORIENTED_EDGE('',*,*,#5530,.F.);
#7843=ORIENTED_EDGE('',*,*,#5590,.T.);
#7844=ORIENTED_EDGE('',*,*,#5597,.F.);
#7845=ORIENTED_EDGE('',*,*,#5600,.F.);
#7846=ORIENTED_EDGE('',*,*,#5598,.F.);
#7847=ORIENTED_EDGE('',*,*,#5601,.T.);
#7848=ORIENTED_EDGE('',*,*,#5602,.T.);
#7849=ORIENTED_EDGE('',*,*,#5600,.T.);
#7850=ORIENTED_EDGE('',*,*,#5603,.T.);
#7851=ORIENTED_EDGE('',*,*,#5604,.T.);
#7852=ORIENTED_EDGE('',*,*,#5605,.T.);
#7853=ORIENTED_EDGE('',*,*,#5594,.T.);
#7854=ORIENTED_EDGE('',*,*,#5606,.T.);
#7855=ORIENTED_EDGE('',*,*,#5607,.T.);
#7856=ORIENTED_EDGE('',*,*,#5601,.F.);
#7857=ORIENTED_EDGE('',*,*,#5596,.F.);
#7858=ORIENTED_EDGE('',*,*,#5607,.F.);
#7859=ORIENTED_EDGE('',*,*,#5520,.F.);
#7860=ORIENTED_EDGE('',*,*,#5541,.F.);
#7861=ORIENTED_EDGE('',*,*,#5521,.F.);
#7862=ORIENTED_EDGE('',*,*,#5606,.F.);
#7863=ORIENTED_EDGE('',*,*,#5592,.F.);
#7864=ORIENTED_EDGE('',*,*,#5608,.T.);
#7865=ORIENTED_EDGE('',*,*,#5566,.T.);
#7866=ORIENTED_EDGE('',*,*,#5609,.T.);
#7867=ORIENTED_EDGE('',*,*,#5609,.F.);
#7868=ORIENTED_EDGE('',*,*,#5568,.F.);
#7869=ORIENTED_EDGE('',*,*,#5605,.F.);
#7870=ORIENTED_EDGE('',*,*,#5610,.F.);
#7871=ORIENTED_EDGE('',*,*,#5549,.F.);
#7872=ORIENTED_EDGE('',*,*,#5564,.F.);
#7873=ORIENTED_EDGE('',*,*,#5608,.F.);
#7874=ORIENTED_EDGE('',*,*,#5611,.F.);
#7875=ORIENTED_EDGE('',*,*,#5551,.F.);
#7876=ORIENTED_EDGE('',*,*,#5612,.F.);
#7877=ORIENTED_EDGE('',*,*,#5604,.F.);
#7878=ORIENTED_EDGE('',*,*,#5569,.F.);
#7879=ORIENTED_EDGE('',*,*,#5559,.T.);
#7880=ORIENTED_EDGE('',*,*,#5570,.F.);
#7881=ORIENTED_EDGE('',*,*,#5603,.F.);
#7882=ORIENTED_EDGE('',*,*,#5567,.F.);
#7883=ORIENTED_EDGE('',*,*,#5531,.F.);
#7884=ORIENTED_EDGE('',*,*,#5599,.F.);
#7885=ORIENTED_EDGE('',*,*,#5602,.F.);
#7886=ORIENTED_EDGE('',*,*,#5519,.F.);
#7887=ORIENTED_EDGE('',*,*,#5611,.T.);
#7888=ORIENTED_EDGE('',*,*,#5610,.T.);
#7889=ORIENTED_EDGE('',*,*,#5612,.T.);
#7890=ORIENTED_EDGE('',*,*,#5550,.F.);
#7891=ORIENTED_EDGE('',*,*,#5613,.F.);
#7892=ORIENTED_EDGE('',*,*,#5614,.F.);
#7893=ORIENTED_EDGE('',*,*,#5615,.F.);
#7894=ORIENTED_EDGE('',*,*,#5616,.F.);
#7895=ORIENTED_EDGE('',*,*,#5617,.F.);
#7896=ORIENTED_EDGE('',*,*,#5618,.F.);
#7897=ORIENTED_EDGE('',*,*,#5619,.F.);
#7898=ORIENTED_EDGE('',*,*,#5620,.F.);
#7899=ORIENTED_EDGE('',*,*,#5621,.F.);
#7900=ORIENTED_EDGE('',*,*,#5613,.T.);
#7901=ORIENTED_EDGE('',*,*,#5622,.T.);
#7902=ORIENTED_EDGE('',*,*,#5620,.T.);
#7903=ORIENTED_EDGE('',*,*,#5623,.T.);
#7904=ORIENTED_EDGE('',*,*,#5539,.T.);
#7905=ORIENTED_EDGE('',*,*,#5624,.T.);
#7906=ORIENTED_EDGE('',*,*,#5621,.T.);
#7907=ORIENTED_EDGE('',*,*,#5625,.T.);
#7908=ORIENTED_EDGE('',*,*,#5626,.F.);
#7909=ORIENTED_EDGE('',*,*,#5627,.F.);
#7910=ORIENTED_EDGE('',*,*,#5628,.F.);
#7911=ORIENTED_EDGE('',*,*,#5627,.T.);
#7912=ORIENTED_EDGE('',*,*,#5629,.T.);
#7913=ORIENTED_EDGE('',*,*,#5617,.T.);
#7914=ORIENTED_EDGE('',*,*,#5630,.T.);
#7915=ORIENTED_EDGE('',*,*,#5619,.T.);
#7916=ORIENTED_EDGE('',*,*,#5631,.T.);
#7917=ORIENTED_EDGE('',*,*,#5628,.T.);
#7918=ORIENTED_EDGE('',*,*,#5632,.T.);
#7919=ORIENTED_EDGE('',*,*,#5537,.T.);
#7920=ORIENTED_EDGE('',*,*,#5633,.T.);
#7921=ORIENTED_EDGE('',*,*,#5626,.T.);
#7922=ORIENTED_EDGE('',*,*,#5634,.T.);
#7923=ORIENTED_EDGE('',*,*,#5535,.T.);
#7924=ORIENTED_EDGE('',*,*,#5635,.T.);
#7925=ORIENTED_EDGE('',*,*,#5618,.T.);
#7926=ORIENTED_EDGE('',*,*,#5636,.T.);
#7927=ORIENTED_EDGE('',*,*,#5616,.T.);
#7928=ORIENTED_EDGE('',*,*,#5637,.T.);
#7929=ORIENTED_EDGE('',*,*,#5614,.T.);
#7930=ORIENTED_EDGE('',*,*,#5638,.T.);
#7931=ORIENTED_EDGE('',*,*,#5533,.T.);
#7932=ORIENTED_EDGE('',*,*,#5639,.T.);
#7933=ORIENTED_EDGE('',*,*,#5615,.T.);
#7934=ORIENTED_EDGE('',*,*,#5640,.T.);
#7935=ORIENTED_EDGE('',*,*,#5634,.F.);
#7936=ORIENTED_EDGE('',*,*,#5631,.F.);
#7937=ORIENTED_EDGE('',*,*,#5624,.F.);
#7938=ORIENTED_EDGE('',*,*,#5538,.F.);
#7939=ORIENTED_EDGE('',*,*,#5456,.T.);
#7940=ORIENTED_EDGE('',*,*,#5540,.F.);
#7941=ORIENTED_EDGE('',*,*,#5625,.F.);
#7942=ORIENTED_EDGE('',*,*,#5622,.F.);
#7943=ORIENTED_EDGE('',*,*,#5639,.F.);
#7944=ORIENTED_EDGE('',*,*,#5532,.F.);
#7945=ORIENTED_EDGE('',*,*,#5472,.T.);
#7946=ORIENTED_EDGE('',*,*,#5485,.T.);
#7947=ORIENTED_EDGE('',*,*,#5630,.F.);
#7948=ORIENTED_EDGE('',*,*,#5638,.F.);
#7949=ORIENTED_EDGE('',*,*,#5623,.F.);
#7950=ORIENTED_EDGE('',*,*,#5632,.F.);
#7951=ORIENTED_EDGE('',*,*,#5446,.T.);
#7952=ORIENTED_EDGE('',*,*,#5442,.T.);
#7953=ORIENTED_EDGE('',*,*,#5440,.T.);
#7954=ORIENTED_EDGE('',*,*,#5437,.T.);
#7955=ORIENTED_EDGE('',*,*,#5434,.T.);
#7956=ORIENTED_EDGE('',*,*,#5432,.T.);
#7957=ORIENTED_EDGE('',*,*,#5635,.F.);
#7958=ORIENTED_EDGE('',*,*,#5534,.F.);
#7959=ORIENTED_EDGE('',*,*,#5640,.F.);
#7960=ORIENTED_EDGE('',*,*,#5637,.F.);
#7961=ORIENTED_EDGE('',*,*,#5633,.F.);
#7962=ORIENTED_EDGE('',*,*,#5536,.F.);
#7963=ORIENTED_EDGE('',*,*,#5636,.F.);
#7964=ORIENTED_EDGE('',*,*,#5629,.F.);
#9213=CYLINDRICAL_SURFACE('',#10262,0.25);
#9214=CYLINDRICAL_SURFACE('',#10264,0.25);
#9215=CYLINDRICAL_SURFACE('',#10266,0.25);
#9216=CYLINDRICAL_SURFACE('',#10268,0.25);
#9217=CYLINDRICAL_SURFACE('',#10274,0.15);
#9218=CYLINDRICAL_SURFACE('',#10276,0.15);
#9219=CYLINDRICAL_SURFACE('',#10279,0.15);
#9220=CYLINDRICAL_SURFACE('',#10282,0.15);
#9221=CYLINDRICAL_SURFACE('',#10284,0.3);
#9222=CYLINDRICAL_SURFACE('',#10289,0.3);
#9223=CYLINDRICAL_SURFACE('',#10294,0.17);
#9224=CYLINDRICAL_SURFACE('',#10296,0.17);
#9225=CYLINDRICAL_SURFACE('',#10320,0.4);
#9226=CYLINDRICAL_SURFACE('',#10321,0.4);
#9227=CYLINDRICAL_SURFACE('',#10344,0.1);
#9228=CYLINDRICAL_SURFACE('',#10348,0.1);
#9229=CYLINDRICAL_SURFACE('',#10362,0.3);
#9230=CYLINDRICAL_SURFACE('',#10367,0.3);
#9555=ADVANCED_FACE('',(#1529),#9213,.F.);
#9556=ADVANCED_FACE('',(#1530),#9214,.F.);
#9557=ADVANCED_FACE('',(#1531),#9215,.F.);
#9558=ADVANCED_FACE('',(#1532),#9216,.F.);
#9559=ADVANCED_FACE('',(#1533),#205,.T.);
#9560=ADVANCED_FACE('',(#1534),#206,.T.);
#9561=ADVANCED_FACE('',(#1535,#147,#148,#149),#1196,.F.);
#9562=ADVANCED_FACE('',(#1536),#9217,.F.);
#9563=ADVANCED_FACE('',(#1537),#9218,.F.);
#9564=ADVANCED_FACE('',(#1538),#9219,.F.);
#9565=ADVANCED_FACE('',(#1539),#9220,.F.);
#9566=ADVANCED_FACE('',(#1540),#9221,.F.);
#9567=ADVANCED_FACE('',(#1541,#150),#1197,.F.);
#9568=ADVANCED_FACE('',(#1542),#9222,.F.);
#9569=ADVANCED_FACE('',(#1543,#151),#1198,.F.);
#9570=ADVANCED_FACE('',(#1544),#9223,.F.);
#9571=ADVANCED_FACE('',(#1545),#9224,.F.);
#9572=ADVANCED_FACE('',(#1546),#1199,.F.);
#9573=ADVANCED_FACE('',(#1547),#1200,.F.);
#9574=ADVANCED_FACE('',(#1548),#1201,.F.);
#9575=ADVANCED_FACE('',(#1549),#1202,.F.);
#9576=ADVANCED_FACE('',(#1550),#1203,.F.);
#9577=ADVANCED_FACE('',(#1551),#1204,.F.);
#9578=ADVANCED_FACE('',(#1552),#1205,.F.);
#9579=ADVANCED_FACE('',(#1553,#152),#1206,.F.);
#9580=ADVANCED_FACE('',(#1554,#153),#1207,.F.);
#9581=ADVANCED_FACE('',(#1555),#1208,.F.);
#9582=ADVANCED_FACE('',(#1556),#1209,.F.);
#9583=ADVANCED_FACE('',(#1557),#1210,.F.);
#9584=ADVANCED_FACE('',(#1558),#1211,.F.);
#9585=ADVANCED_FACE('',(#1559),#1212,.F.);
#9586=ADVANCED_FACE('',(#1560),#1213,.T.);
#9587=ADVANCED_FACE('',(#1561),#1214,.T.);
#9588=ADVANCED_FACE('',(#1562),#1215,.T.);
#9589=ADVANCED_FACE('',(#1563),#1216,.T.);
#9590=ADVANCED_FACE('',(#1564),#1217,.T.);
#9591=ADVANCED_FACE('',(#1565,#154),#1218,.F.);
#9592=ADVANCED_FACE('',(#1566),#9225,.T.);
#9593=ADVANCED_FACE('',(#1567),#9226,.T.);
#9594=ADVANCED_FACE('',(#1568),#1219,.T.);
#9595=ADVANCED_FACE('',(#1569),#207,.T.);
#9596=ADVANCED_FACE('',(#1570),#208,.T.);
#9597=ADVANCED_FACE('',(#1571),#209,.T.);
#9598=ADVANCED_FACE('',(#1572),#210,.T.);
#9599=ADVANCED_FACE('',(#1573),#1220,.F.);
#9600=ADVANCED_FACE('',(#1574),#211,.T.);
#9601=ADVANCED_FACE('',(#1575),#212,.T.);
#9602=ADVANCED_FACE('',(#1576),#1221,.T.);
#9603=ADVANCED_FACE('',(#1577),#213,.T.);
#9604=ADVANCED_FACE('',(#1578),#214,.T.);
#9605=ADVANCED_FACE('',(#1579),#1222,.F.);
#9606=ADVANCED_FACE('',(#1580),#215,.T.);
#9607=ADVANCED_FACE('',(#1581),#216,.T.);
#9608=ADVANCED_FACE('',(#1582),#1223,.T.);
#9609=ADVANCED_FACE('',(#1583),#217,.T.);
#9610=ADVANCED_FACE('',(#1584),#218,.T.);
#9611=ADVANCED_FACE('',(#1585,#155,#156,#157),#1224,.F.);
#9612=ADVANCED_FACE('',(#1586),#219,.T.);
#9613=ADVANCED_FACE('',(#1587),#1225,.T.);
#9614=ADVANCED_FACE('',(#1588),#220,.T.);
#9615=ADVANCED_FACE('',(#1589),#221,.T.);
#9616=ADVANCED_FACE('',(#1590),#1226,.F.);
#9617=ADVANCED_FACE('',(#1591),#222,.T.);
#9618=ADVANCED_FACE('',(#1592),#223,.T.);
#9619=ADVANCED_FACE('',(#1593),#76,.F.);
#9620=ADVANCED_FACE('',(#1594),#77,.F.);
#9621=ADVANCED_FACE('',(#1595),#78,.F.);
#9622=ADVANCED_FACE('',(#1596),#9227,.F.);
#9623=ADVANCED_FACE('',(#1597),#224,.T.);
#9624=ADVANCED_FACE('',(#1598),#79,.F.);
#9625=ADVANCED_FACE('',(#1599),#9228,.F.);
#9626=ADVANCED_FACE('',(#1600),#225,.T.);
#9627=ADVANCED_FACE('',(#1601),#226,.T.);
#9628=ADVANCED_FACE('',(#1602),#227,.T.);
#9629=ADVANCED_FACE('',(#1603),#228,.T.);
#9630=ADVANCED_FACE('',(#1604),#1227,.T.);
#9631=ADVANCED_FACE('',(#1605),#80,.T.);
#9632=ADVANCED_FACE('',(#1606),#81,.T.);
#9633=ADVANCED_FACE('',(#1607),#82,.T.);
#9634=ADVANCED_FACE('',(#1608),#9229,.T.);
#9635=ADVANCED_FACE('',(#1609),#229,.F.);
#9636=ADVANCED_FACE('',(#1610),#83,.T.);
#9637=ADVANCED_FACE('',(#1611),#9230,.T.);
#9638=ADVANCED_FACE('',(#1612),#230,.F.);
#9639=ADVANCED_FACE('',(#1613),#231,.F.);
#9640=ADVANCED_FACE('',(#1614),#232,.F.);
#9641=ADVANCED_FACE('',(#1615),#233,.F.);
#9642=ADVANCED_FACE('',(#1616),#234,.F.);
#9643=ADVANCED_FACE('',(#1617),#235,.F.);
#9644=ADVANCED_FACE('',(#1618),#1228,.F.);
#9645=ADVANCED_FACE('',(#1619,#158,#159,#160,#161,#162,#163),#1229,.T.);
#9646=ADVANCED_FACE('',(#1620),#236,.F.);
#9647=ADVANCED_FACE('',(#1621),#1230,.F.);
#9893=CLOSED_SHELL('',(#9555,#9556,#9557,#9558,#9559,#9560,#9561,#9562,
#9563,#9564,#9565,#9566,#9567,#9568,#9569,#9570,#9571,#9572,#9573,#9574,
#9575,#9576,#9577,#9578,#9579,#9580,#9581,#9582,#9583,#9584,#9585,#9586,
#9587,#9588,#9589,#9590,#9591,#9592,#9593,#9594,#9595,#9596,#9597,#9598,
#9599,#9600,#9601,#9602,#9603,#9604,#9605,#9606,#9607,#9608,#9609,#9610,
#9611,#9612,#9613,#9614,#9615,#9616,#9617,#9618,#9619,#9620,#9621,#9622,
#9623,#9624,#9625,#9626,#9627,#9628,#9629,#9630,#9631,#9632,#9633,#9634,
#9635,#9636,#9637,#9638,#9639,#9640,#9641,#9642,#9643,#9644,#9645,#9646,
#9647));
#10261=AXIS2_PLACEMENT_3D('',#14938,#11431,#11432);
#10262=AXIS2_PLACEMENT_3D('',#14939,#11433,#11434);
#10263=AXIS2_PLACEMENT_3D('',#14966,#11435,#11436);
#10264=AXIS2_PLACEMENT_3D('',#14967,#11437,#11438);
#10265=AXIS2_PLACEMENT_3D('',#14990,#11439,#11440);
#10266=AXIS2_PLACEMENT_3D('',#14991,#11441,#11442);
#10267=AXIS2_PLACEMENT_3D('',#15014,#11443,#11444);
#10268=AXIS2_PLACEMENT_3D('',#15015,#11445,#11446);
#10269=AXIS2_PLACEMENT_3D('',#15042,#11447,#11448);
#10270=AXIS2_PLACEMENT_3D('',#15227,#11449,#11450);
#10271=AXIS2_PLACEMENT_3D('',#15241,#11453,#11454);
#10272=AXIS2_PLACEMENT_3D('',#15243,#11455,#11456);
#10273=AXIS2_PLACEMENT_3D('',#15245,#11457,#11458);
#10274=AXIS2_PLACEMENT_3D('',#15246,#11459,#11460);
#10275=AXIS2_PLACEMENT_3D('',#15248,#11461,#11462);
#10276=AXIS2_PLACEMENT_3D('',#15250,#11464,#11465);
#10277=AXIS2_PLACEMENT_3D('',#15252,#11466,#11467);
#10278=AXIS2_PLACEMENT_3D('',#15255,#11469,#11470);
#10279=AXIS2_PLACEMENT_3D('',#15256,#11471,#11472);
#10280=AXIS2_PLACEMENT_3D('',#15258,#11473,#11474);
#10281=AXIS2_PLACEMENT_3D('',#15261,#11476,#11477);
#10282=AXIS2_PLACEMENT_3D('',#15262,#11478,#11479);
#10283=AXIS2_PLACEMENT_3D('',#15264,#11480,#11481);
#10284=AXIS2_PLACEMENT_3D('',#15266,#11483,#11484);
#10285=AXIS2_PLACEMENT_3D('',#15268,#11485,#11486);
#10286=AXIS2_PLACEMENT_3D('',#15271,#11488,#11489);
#10287=AXIS2_PLACEMENT_3D('',#15272,#11490,#11491);
#10288=AXIS2_PLACEMENT_3D('',#15274,#11492,#11493);
#10289=AXIS2_PLACEMENT_3D('',#15275,#11494,#11495);
#10290=AXIS2_PLACEMENT_3D('',#15277,#11496,#11497);
#10291=AXIS2_PLACEMENT_3D('',#15280,#11499,#11500);
#10292=AXIS2_PLACEMENT_3D('',#15281,#11501,#11502);
#10293=AXIS2_PLACEMENT_3D('',#15283,#11503,#11504);
#10294=AXIS2_PLACEMENT_3D('',#15284,#11505,#11506);
#10295=AXIS2_PLACEMENT_3D('',#15287,#11508,#11509);
#10296=AXIS2_PLACEMENT_3D('',#15288,#11510,#11511);
#10297=AXIS2_PLACEMENT_3D('',#15291,#11513,#11514);
#10298=AXIS2_PLACEMENT_3D('',#15292,#11515,#11516);
#10299=AXIS2_PLACEMENT_3D('',#15301,#11521,#11522);
#10300=AXIS2_PLACEMENT_3D('',#15310,#11527,#11528);
#10301=AXIS2_PLACEMENT_3D('',#15319,#11533,#11534);
#10302=AXIS2_PLACEMENT_3D('',#15328,#11539,#11540);
#10303=AXIS2_PLACEMENT_3D('',#15337,#11545,#11546);
#10304=AXIS2_PLACEMENT_3D('',#15346,#11551,#11552);
#10305=AXIS2_PLACEMENT_3D('',#15355,#11557,#11558);
#10306=AXIS2_PLACEMENT_3D('',#15357,#11559,#11560);
#10307=AXIS2_PLACEMENT_3D('',#15358,#11561,#11562);
#10308=AXIS2_PLACEMENT_3D('',#15360,#11563,#11564);
#10309=AXIS2_PLACEMENT_3D('',#15361,#11565,#11566);
#10310=AXIS2_PLACEMENT_3D('',#15364,#11569,#11570);
#10311=AXIS2_PLACEMENT_3D('',#15367,#11573,#11574);
#10312=AXIS2_PLACEMENT_3D('',#15370,#11577,#11578);
#10313=AXIS2_PLACEMENT_3D('',#15376,#11582,#11583);
#10314=AXIS2_PLACEMENT_3D('',#15382,#11587,#11588);
#10315=AXIS2_PLACEMENT_3D('',#15427,#11590,#11591);
#10316=AXIS2_PLACEMENT_3D('',#15473,#11594,#11595);
#10317=AXIS2_PLACEMENT_3D('',#15551,#11599,#11600);
#10318=AXIS2_PLACEMENT_3D('',#15599,#11604,#11605);
#10319=AXIS2_PLACEMENT_3D('',#15615,#11609,#11610);
#10320=AXIS2_PLACEMENT_3D('',#15936,#11622,#11623);
#10321=AXIS2_PLACEMENT_3D('',#15938,#11625,#11626);
#10322=AXIS2_PLACEMENT_3D('',#15940,#11627,#11628);
#10323=AXIS2_PLACEMENT_3D('',#15942,#11630,#11631);
#10324=AXIS2_PLACEMENT_3D('',#16106,#11633,#11634);
#10325=AXIS2_PLACEMENT_3D('',#16107,#11635,#11636);
#10326=AXIS2_PLACEMENT_3D('',#16155,#11638,#11639);
#10327=AXIS2_PLACEMENT_3D('',#16273,#11641,#11642);
#10328=AXIS2_PLACEMENT_3D('',#16318,#11643,#11644);
#10329=AXIS2_PLACEMENT_3D('',#16410,#11646,#11647);
#10330=AXIS2_PLACEMENT_3D('',#16427,#11648,#11649);
#10331=AXIS2_PLACEMENT_3D('',#16547,#11651,#11652);
#10332=AXIS2_PLACEMENT_3D('',#16552,#11653,#11654);
#10333=AXIS2_PLACEMENT_3D('',#16604,#11656,#11657);
#10334=AXIS2_PLACEMENT_3D('',#16605,#11658,#11659);
#10335=AXIS2_PLACEMENT_3D('',#16606,#11660,#11661);
#10336=AXIS2_PLACEMENT_3D('',#16607,#11662,#11663);
#10337=AXIS2_PLACEMENT_3D('',#16608,#11664,#11665);
#10338=AXIS2_PLACEMENT_3D('',#16609,#11666,#11667);
#10339=AXIS2_PLACEMENT_3D('',#16611,#11668,#11669);
#10340=AXIS2_PLACEMENT_3D('',#16612,#11670,#11671);
#10341=AXIS2_PLACEMENT_3D('',#16613,#11672,#11673);
#10342=AXIS2_PLACEMENT_3D('',#16614,#11674,#11675);
#10343=AXIS2_PLACEMENT_3D('',#16615,#11676,#11677);
#10344=AXIS2_PLACEMENT_3D('',#16616,#11678,#11679);
#10345=AXIS2_PLACEMENT_3D('',#16637,#11680,#11681);
#10346=AXIS2_PLACEMENT_3D('',#16639,#11682,#11683);
#10347=AXIS2_PLACEMENT_3D('',#16640,#11684,#11685);
#10348=AXIS2_PLACEMENT_3D('',#16641,#11686,#11687);
#10349=AXIS2_PLACEMENT_3D('',#16731,#11689,#11690);
#10350=AXIS2_PLACEMENT_3D('',#16732,#11691,#11692);
#10351=AXIS2_PLACEMENT_3D('',#16735,#11693,#11694);
#10352=AXIS2_PLACEMENT_3D('',#16737,#11695,#11696);
#10353=AXIS2_PLACEMENT_3D('',#16738,#11697,#11698);
#10354=AXIS2_PLACEMENT_3D('',#16739,#11699,#11700);
#10355=AXIS2_PLACEMENT_3D('',#16742,#11701,#11702);
#10356=AXIS2_PLACEMENT_3D('',#16744,#11703,#11704);
#10357=AXIS2_PLACEMENT_3D('',#16745,#11705,#11706);
#10358=AXIS2_PLACEMENT_3D('',#16746,#11707,#11708);
#10359=AXIS2_PLACEMENT_3D('',#16749,#11709,#11710);
#10360=AXIS2_PLACEMENT_3D('',#16751,#11711,#11712);
#10361=AXIS2_PLACEMENT_3D('',#16752,#11713,#11714);
#10362=AXIS2_PLACEMENT_3D('',#16753,#11715,#11716);
#10363=AXIS2_PLACEMENT_3D('',#16784,#11719,#11720);
#10364=AXIS2_PLACEMENT_3D('',#16787,#11721,#11722);
#10365=AXIS2_PLACEMENT_3D('',#16789,#11723,#11724);
#10366=AXIS2_PLACEMENT_3D('',#16790,#11725,#11726);
#10367=AXIS2_PLACEMENT_3D('',#16791,#11727,#11728);
#10368=AXIS2_PLACEMENT_3D('',#16964,#11731,#11732);
#10369=AXIS2_PLACEMENT_3D('',#16965,#11733,#11734);
#10370=AXIS2_PLACEMENT_3D('',#16982,#11735,#11736);
#11431=DIRECTION('axis',(0.,0.,1.));
#11432=DIRECTION('refdir',(1.,0.,0.));
#11433=DIRECTION('center_axis',(0.,0.,-1.));
#11434=DIRECTION('ref_axis',(1.,0.,0.));
#11435=DIRECTION('center_axis',(0.,0.,1.));
#11436=DIRECTION('ref_axis',(1.,0.,0.));
#11437=DIRECTION('center_axis',(0.,0.,-1.));
#11438=DIRECTION('ref_axis',(1.,0.,0.));
#11439=DIRECTION('center_axis',(0.,0.,1.));
#11440=DIRECTION('ref_axis',(1.,0.,0.));
#11441=DIRECTION('center_axis',(0.,0.,-1.));
#11442=DIRECTION('ref_axis',(1.,0.,0.));
#11443=DIRECTION('center_axis',(0.,0.,1.));
#11444=DIRECTION('ref_axis',(1.,0.,0.));
#11445=DIRECTION('center_axis',(0.,0.,-1.));
#11446=DIRECTION('ref_axis',(1.,0.,0.));
#11447=DIRECTION('center_axis',(0.,0.,1.));
#11448=DIRECTION('ref_axis',(1.,0.,0.));
#11449=DIRECTION('center_axis',(4.10828654779316E-33,-1.13946463231163E-19,
1.));
#11450=DIRECTION('ref_axis',(1.,0.,-4.10828654779316E-33));
#11451=DIRECTION('',(0.,1.,1.13946463231163E-19));
#11452=DIRECTION('',(0.,-1.,-1.13946463231163E-19));
#11453=DIRECTION('center_axis',(4.10828654779316E-33,-1.13946463231163E-19,
1.));
#11454=DIRECTION('ref_axis',(1.,0.,0.));
#11455=DIRECTION('center_axis',(4.10828654779316E-33,-1.13946463231163E-19,
1.));
#11456=DIRECTION('ref_axis',(1.,0.,0.));
#11457=DIRECTION('center_axis',(4.10828654779316E-33,-1.13946463231163E-19,
1.));
#11458=DIRECTION('ref_axis',(1.,0.,0.));
#11459=DIRECTION('center_axis',(0.,0.,-1.));
#11460=DIRECTION('ref_axis',(1.,0.,0.));
#11461=DIRECTION('center_axis',(-4.10828654779316E-33,1.13946463231163E-19,
-1.));
#11462=DIRECTION('ref_axis',(1.,0.,0.));
#11463=DIRECTION('',(0.,0.,-1.));
#11464=DIRECTION('center_axis',(0.,0.,-1.));
#11465=DIRECTION('ref_axis',(1.,0.,0.));
#11466=DIRECTION('center_axis',(-4.10828654779316E-33,1.13946463231163E-19,
-1.));
#11467=DIRECTION('ref_axis',(1.,0.,0.));
#11468=DIRECTION('',(0.,0.,-1.));
#11469=DIRECTION('center_axis',(4.10828654779316E-33,-1.13946463231163E-19,
1.));
#11470=DIRECTION('ref_axis',(1.,0.,0.));
#11471=DIRECTION('center_axis',(0.,0.,-1.));
#11472=DIRECTION('ref_axis',(1.,0.,0.));
#11473=DIRECTION('center_axis',(-4.10828654779316E-33,1.13946463231163E-19,
-1.));
#11474=DIRECTION('ref_axis',(1.,0.,0.));
#11475=DIRECTION('',(0.,0.,-1.));
#11476=DIRECTION('center_axis',(4.10828654779316E-33,-1.13946463231163E-19,
1.));
#11477=DIRECTION('ref_axis',(1.,0.,0.));
#11478=DIRECTION('center_axis',(0.,0.,-1.));
#11479=DIRECTION('ref_axis',(1.,0.,0.));
#11480=DIRECTION('center_axis',(-4.10828654779316E-33,1.13946463231163E-19,
-1.));
#11481=DIRECTION('ref_axis',(1.,0.,0.));
#11482=DIRECTION('',(0.,0.,-1.));
#11483=DIRECTION('center_axis',(0.,0.,-1.));
#11484=DIRECTION('ref_axis',(1.,0.,0.));
#11485=DIRECTION('center_axis',(-4.10828654779316E-33,1.13946463231163E-19,
-1.));
#11486=DIRECTION('ref_axis',(1.,0.,0.));
#11487=DIRECTION('',(0.,0.,-1.));
#11488=DIRECTION('center_axis',(0.,0.,-1.));
#11489=DIRECTION('ref_axis',(1.,0.,0.));
#11490=DIRECTION('center_axis',(0.,0.,-1.));
#11491=DIRECTION('ref_axis',(1.,0.,0.));
#11492=DIRECTION('center_axis',(0.,0.,1.));
#11493=DIRECTION('ref_axis',(1.,0.,0.));
#11494=DIRECTION('center_axis',(0.,0.,-1.));
#11495=DIRECTION('ref_axis',(1.,0.,0.));
#11496=DIRECTION('center_axis',(-4.10828654779316E-33,1.13946463231163E-19,
-1.));
#11497=DIRECTION('ref_axis',(1.,0.,0.));
#11498=DIRECTION('',(0.,0.,-1.));
#11499=DIRECTION('center_axis',(0.,0.,-1.));
#11500=DIRECTION('ref_axis',(1.,0.,0.));
#11501=DIRECTION('center_axis',(0.,0.,-1.));
#11502=DIRECTION('ref_axis',(1.,0.,0.));
#11503=DIRECTION('center_axis',(0.,0.,1.));
#11504=DIRECTION('ref_axis',(1.,0.,0.));
#11505=DIRECTION('center_axis',(0.,0.,-1.));
#11506=DIRECTION('ref_axis',(1.,0.,0.));
#11507=DIRECTION('',(0.,0.,-1.));
#11508=DIRECTION('center_axis',(0.,0.,1.));
#11509=DIRECTION('ref_axis',(1.,0.,0.));
#11510=DIRECTION('center_axis',(0.,0.,-1.));
#11511=DIRECTION('ref_axis',(1.,0.,0.));
#11512=DIRECTION('',(0.,0.,-1.));
#11513=DIRECTION('center_axis',(0.,0.,1.));
#11514=DIRECTION('ref_axis',(1.,0.,0.));
#11515=DIRECTION('center_axis',(0.,-1.,0.));
#11516=DIRECTION('ref_axis',(-1.,0.,0.));
#11517=DIRECTION('',(0.0523359562429438,0.,0.998629534754574));
#11518=DIRECTION('',(1.,0.,0.));
#11519=DIRECTION('',(-0.0523359562429438,0.,-0.998629534754574));
#11520=DIRECTION('',(1.,0.,0.));
#11521=DIRECTION('center_axis',(0.,-1.,0.));
#11522=DIRECTION('ref_axis',(-1.,0.,0.));
#11523=DIRECTION('',(0.,0.,-1.));
#11524=DIRECTION('',(1.,0.,0.));
#11525=DIRECTION('',(0.,0.,1.));
#11526=DIRECTION('',(1.,0.,0.));
#11527=DIRECTION('center_axis',(0.,-1.,0.));
#11528=DIRECTION('ref_axis',(-1.,0.,0.));
#11529=DIRECTION('',(0.,0.,-1.));
#11530=DIRECTION('',(1.,0.,0.));
#11531=DIRECTION('',(0.,0.,1.));
#11532=DIRECTION('',(1.,0.,0.));
#11533=DIRECTION('center_axis',(0.,-1.,0.));
#11534=DIRECTION('ref_axis',(-1.,0.,0.));
#11535=DIRECTION('',(0.,0.,-1.));
#11536=DIRECTION('',(1.,0.,0.));
#11537=DIRECTION('',(0.,0.,1.));
#11538=DIRECTION('',(1.,0.,0.));
#11539=DIRECTION('center_axis',(0.,1.,0.));
#11540=DIRECTION('ref_axis',(1.,0.,0.));
#11541=DIRECTION('',(-0.0523359562429438,0.,-0.998629534754574));
#11542=DIRECTION('',(-1.,0.,0.));
#11543=DIRECTION('',(0.0523359562429438,0.,0.998629534754574));
#11544=DIRECTION('',(-1.,0.,0.));
#11545=DIRECTION('center_axis',(0.,1.,0.));
#11546=DIRECTION('ref_axis',(1.,0.,0.));
#11547=DIRECTION('',(0.,0.,1.));
#11548=DIRECTION('',(-1.,0.,0.));
#11549=DIRECTION('',(0.,0.,-1.));
#11550=DIRECTION('',(-1.,0.,0.));
#11551=DIRECTION('center_axis',(0.,1.,0.));
#11552=DIRECTION('ref_axis',(1.,0.,0.));
#11553=DIRECTION('',(0.,0.,1.));
#11554=DIRECTION('',(-1.,0.,0.));
#11555=DIRECTION('',(0.,0.,-1.));
#11556=DIRECTION('',(-1.,0.,0.));
#11557=DIRECTION('center_axis',(0.,0.,1.));
#11558=DIRECTION('ref_axis',(1.,0.,0.));
#11559=DIRECTION('center_axis',(0.,0.,1.));
#11560=DIRECTION('ref_axis',(1.,0.,0.));
#11561=DIRECTION('center_axis',(0.,0.,1.));
#11562=DIRECTION('ref_axis',(1.,0.,0.));
#11563=DIRECTION('center_axis',(0.,0.,1.));
#11564=DIRECTION('ref_axis',(1.,0.,0.));
#11565=DIRECTION('center_axis',(0.,0.,1.));
#11566=DIRECTION('ref_axis',(1.,0.,0.));
#11567=DIRECTION('',(0.,1.,0.));
#11568=DIRECTION('',(0.,-1.,0.));
#11569=DIRECTION('center_axis',(0.,0.,1.));
#11570=DIRECTION('ref_axis',(1.,0.,0.));
#11571=DIRECTION('',(0.,-1.,0.));
#11572=DIRECTION('',(0.,1.,0.));
#11573=DIRECTION('center_axis',(0.,0.,1.));
#11574=DIRECTION('ref_axis',(1.,0.,0.));
#11575=DIRECTION('',(0.,-1.,0.));
#11576=DIRECTION('',(0.,1.,0.));
#11577=DIRECTION('center_axis',(0.,0.,1.));
#11578=DIRECTION('ref_axis',(1.,0.,0.));
#11579=DIRECTION('',(0.,-1.,0.));
#11580=DIRECTION('',(-1.,0.,0.));
#11581=DIRECTION('',(0.,1.,0.));
#11582=DIRECTION('center_axis',(0.,1.,0.));
#11583=DIRECTION('ref_axis',(1.,0.,0.));
#11584=DIRECTION('',(0.,0.,1.));
#11585=DIRECTION('',(-1.,0.,0.));
#11586=DIRECTION('',(0.,0.,-1.));
#11587=DIRECTION('center_axis',(-1.,0.,0.));
#11588=DIRECTION('ref_axis',(0.,-1.,0.));
#11589=DIRECTION('',(0.,-1.,0.));
#11590=DIRECTION('center_axis',(1.,0.,0.));
#11591=DIRECTION('ref_axis',(0.,1.,0.));
#11592=DIRECTION('',(0.,1.,0.));
#11593=DIRECTION('',(0.,1.,0.));
#11594=DIRECTION('center_axis',(1.,0.,0.));
#11595=DIRECTION('ref_axis',(0.,1.,0.));
#11596=DIRECTION('',(0.,1.,0.));
#11597=DIRECTION('',(0.,1.,1.13946463231163E-19));
#11598=DIRECTION('',(0.,1.,0.));
#11599=DIRECTION('center_axis',(1.,0.,0.));
#11600=DIRECTION('ref_axis',(0.,1.,0.));
#11601=DIRECTION('',(0.,1.,0.));
#11602=DIRECTION('',(0.,1.,1.13946463231163E-19));
#11603=DIRECTION('',(0.,1.,0.));
#11604=DIRECTION('center_axis',(0.998629534754574,0.,-0.0523359562429438));
#11605=DIRECTION('ref_axis',(-0.0523359562429438,0.,-0.998629534754574));
#11606=DIRECTION('',(0.,-1.,0.));
#11607=DIRECTION('',(-5.97168109510197E-21,-1.,-1.13946463231163E-19));
#11608=DIRECTION('',(0.,-1.,0.));
#11609=DIRECTION('center_axis',(0.,0.,1.));
#11610=DIRECTION('ref_axis',(1.,0.,0.));
#11611=DIRECTION('',(0.,-1.,0.));
#11612=DIRECTION('',(0.,-1.,0.));
#11613=DIRECTION('',(0.,-1.,0.));
#11614=DIRECTION('',(0.,1.,0.));
#11615=DIRECTION('',(0.,-1.,0.));
#11616=DIRECTION('',(0.,1.,0.));
#11617=DIRECTION('',(0.,-1.,0.));
#11618=DIRECTION('',(0.,-1.,0.));
#11619=DIRECTION('',(0.,-1.,0.));
#11620=DIRECTION('',(0.,1.,0.));
#11621=DIRECTION('',(0.,1.,0.));
#11622=DIRECTION('center_axis',(0.,0.,1.));
#11623=DIRECTION('ref_axis',(1.,0.,0.));
#11624=DIRECTION('',(0.,0.,-1.));
#11625=DIRECTION('center_axis',(0.,0.,1.));
#11626=DIRECTION('ref_axis',(1.,0.,0.));
#11627=DIRECTION('center_axis',(4.10828654779316E-33,-1.13946463231163E-19,
1.));
#11628=DIRECTION('ref_axis',(1.,0.,0.));
#11629=DIRECTION('',(0.,0.,-1.));
#11630=DIRECTION('center_axis',(1.,0.,0.));
#11631=DIRECTION('ref_axis',(0.,1.,0.));
#11632=DIRECTION('',(0.,1.,1.13946463231163E-19));
#11633=DIRECTION('center_axis',(0.99852593895705,0.0542765992849681,9.38276897523041E-9));
#11634=DIRECTION('ref_axis',(0.0541946171271057,-0.99701772369063,0.0549418066794405));
#11635=DIRECTION('center_axis',(4.10828654779316E-33,-1.13946463231163E-19,
1.));
#11636=DIRECTION('ref_axis',(1.,0.,-4.10828654779316E-33));
#11637=DIRECTION('',(5.97168109510217E-21,-1.,-1.13946463231163E-19));
#11638=DIRECTION('center_axis',(-1.,0.,0.));
#11639=DIRECTION('ref_axis',(0.,-1.,0.));
#11640=DIRECTION('',(0.,-1.,-1.13946463231163E-19));
#11641=DIRECTION('center_axis',(4.10828654779316E-33,-1.13946463231163E-19,
1.));
#11642=DIRECTION('ref_axis',(1.,0.,-4.10828654779316E-33));
#11643=DIRECTION('center_axis',(-1.,0.,0.));
#11644=DIRECTION('ref_axis',(0.,-1.,0.));
#11645=DIRECTION('',(0.,-1.,-1.13946463231163E-19));
#11646=DIRECTION('center_axis',(4.10828654779316E-33,-1.13946463231163E-19,
1.));
#11647=DIRECTION('ref_axis',(1.,0.,-4.10828654779316E-33));
#11648=DIRECTION('center_axis',(-1.,0.,0.));
#11649=DIRECTION('ref_axis',(0.,-1.,0.));
#11650=DIRECTION('',(0.,-1.,-1.13946463231163E-19));
#11651=DIRECTION('center_axis',(-0.996961060527779,0.0779015005717205,0.));
#11652=DIRECTION('ref_axis',(0.,0.,1.));
#11653=DIRECTION('center_axis',(4.10828654779316E-33,-1.13946463231163E-19,
1.));
#11654=DIRECTION('ref_axis',(1.,0.,-4.10828654779316E-33));
#11655=DIRECTION('',(5.97168109510197E-21,1.,1.13946463231163E-19));
#11656=DIRECTION('center_axis',(-0.996961060527779,-0.0779015005717276,
-4.485055189269E-15));
#11657=DIRECTION('ref_axis',(-0.0777791112471086,0.995394757055134,0.0560329142626144));
#11658=DIRECTION('center_axis',(-0.377317868652411,-0.840644185582845,0.388521015186253));
#11659=DIRECTION('ref_axis',(-0.58566693710526,0.541587807512093,0.603056287203763));
#11660=DIRECTION('center_axis',(7.41164423166535E-16,1.,0.));
#11661=DIRECTION('ref_axis',(0.,0.,1.));
#11662=DIRECTION('center_axis',(0.0522650005536027,-0.0520548592672972,
0.997275619547472));
#11663=DIRECTION('ref_axis',(-0.998629534754574,7.40148683083438E-16,0.0523359562429445));
#11664=DIRECTION('center_axis',(0.376559988603802,-0.837471124372148,0.396036224133039));
#11665=DIRECTION('ref_axis',(0.577069986161316,0.546481578685729,0.606916893181374));
#11666=DIRECTION('center_axis',(0.998525938475037,-0.0542766081525538,0.));
#11667=DIRECTION('ref_axis',(0.,0.,1.));
#11668=DIRECTION('center_axis',(-0.0522648366634829,-0.0521149007022807,
0.997272492337641));
#11669=DIRECTION('ref_axis',(0.0541946171271058,0.99701772369063,0.0549418066794413));
#11670=DIRECTION('center_axis',(5.32220538281047E-11,1.,-1.01553728389566E-9));
#11671=DIRECTION('ref_axis',(0.998629534754574,0.,0.0523359562429456));
#11672=DIRECTION('center_axis',(0.37731786865241,-0.840644185582843,-0.388521015186259));
#11673=DIRECTION('ref_axis',(-0.585666937105255,-0.541587807512096,0.603056287203765));
#11674=DIRECTION('center_axis',(0.0522650005536027,0.0520548592672965,0.997275619547472));
#11675=DIRECTION('ref_axis',(-0.0777791112471059,-0.995394757055134,0.0560329142626137));
#11676=DIRECTION('center_axis',(0.,-1.,0.));
#11677=DIRECTION('ref_axis',(-0.998629534754574,0.,0.0523359562429439));
#11678=DIRECTION('center_axis',(5.97168109510197E-21,1.,1.13946463231163E-19));
#11679=DIRECTION('ref_axis',(-0.688354575693753,0.,0.725374371012288));
#11680=DIRECTION('center_axis',(-0.376559987018669,-0.837471124206646,-0.396036225990193));
#11681=DIRECTION('ref_axis',(0.577069983350267,-0.54648157893936,0.606916895625808));
#11682=DIRECTION('center_axis',(-0.0522648366634817,0.0521149007022785,
0.997272492337641));
#11683=DIRECTION('ref_axis',(0.998629534754574,0.,0.052335956242946));
#11684=DIRECTION('center_axis',(1.01693095242295E-9,-1.,0.));
#11685=DIRECTION('ref_axis',(0.,0.,1.));
#11686=DIRECTION('center_axis',(5.97168109510217E-21,-1.,-1.13946463231163E-19));
#11687=DIRECTION('ref_axis',(0.688354575693753,0.,0.725374371012289));
#11688=DIRECTION('',(-5.97168109510217E-21,1.,1.13946463231163E-19));
#11689=DIRECTION('center_axis',(-0.998629534754574,0.,-0.0523359562429455));
#11690=DIRECTION('ref_axis',(-0.0523359562429455,0.,0.998629534754574));
#11691=DIRECTION('center_axis',(-0.377317868652411,-0.840644185582845,0.388521015186254));
#11692=DIRECTION('ref_axis',(-0.585666937105261,0.541587807512092,0.603056287203763));
#11693=DIRECTION('center_axis',(7.41164423166535E-16,1.,0.));
#11694=DIRECTION('ref_axis',(0.,0.,1.));
#11695=DIRECTION('center_axis',(-0.996961060527779,-0.0779015005717276,
-4.485055189269E-15));
#11696=DIRECTION('ref_axis',(-0.0777791112471086,0.995394757055134,0.0560329142626144));
#11697=DIRECTION('center_axis',(0.0522650005536027,-0.0520548592672972,
0.997275619547472));
#11698=DIRECTION('ref_axis',(-0.998629534754574,7.40148683083438E-16,0.0523359562429445));
#11699=DIRECTION('center_axis',(0.376559988603802,-0.837471124372148,0.396036224133039));
#11700=DIRECTION('ref_axis',(0.577069986161311,0.546481578685732,0.606916893181376));
#11701=DIRECTION('center_axis',(0.998525938475037,-0.0542766081525538,0.));
#11702=DIRECTION('ref_axis',(0.,0.,1.));
#11703=DIRECTION('center_axis',(5.32220538281047E-11,1.,-1.01553728389566E-9));
#11704=DIRECTION('ref_axis',(0.998629534754574,0.,0.0523359562429456));
#11705=DIRECTION('center_axis',(-0.0522648366634829,-0.0521149007022807,
0.997272492337641));
#11706=DIRECTION('ref_axis',(0.0541946171271058,0.99701772369063,0.0549418066794413));
#11707=DIRECTION('center_axis',(0.37731786865241,-0.840644185582843,-0.388521015186259));
#11708=DIRECTION('ref_axis',(-0.585666937105255,-0.541587807512095,0.603056287203766));
#11709=DIRECTION('center_axis',(-0.996961060527779,0.0779015005717205,0.));
#11710=DIRECTION('ref_axis',(0.,0.,1.));
#11711=DIRECTION('center_axis',(0.,-1.,0.));
#11712=DIRECTION('ref_axis',(-0.998629534754574,0.,0.0523359562429439));
#11713=DIRECTION('center_axis',(0.0522650005536027,0.0520548592672965,0.997275619547472));
#11714=DIRECTION('ref_axis',(-0.0777791112471059,-0.995394757055134,0.0560329142626137));
#11715=DIRECTION('center_axis',(5.97168109510197E-21,1.,1.13946463231163E-19));
#11716=DIRECTION('ref_axis',(-0.688354575693753,0.,0.725374371012289));
#11717=DIRECTION('',(-5.97168109510197E-21,-1.,-1.13946463231163E-19));
#11718=DIRECTION('',(5.97168109510197E-21,1.,1.13946463231163E-19));
#11719=DIRECTION('center_axis',(-0.376559987018669,-0.837471124206646,-0.396036225990194));
#11720=DIRECTION('ref_axis',(0.577069983350267,-0.546481578939359,0.606916895625808));
#11721=DIRECTION('center_axis',(-0.0522648366634817,0.0521149007022785,
0.997272492337641));
#11722=DIRECTION('ref_axis',(0.998629534754574,0.,0.052335956242946));
#11723=DIRECTION('center_axis',(1.01693095242295E-9,-1.,0.));
#11724=DIRECTION('ref_axis',(0.,0.,1.));
#11725=DIRECTION('center_axis',(0.99852593895705,0.0542765992849681,9.38276897523041E-9));
#11726=DIRECTION('ref_axis',(0.0541946171271057,-0.99701772369063,0.0549418066794405));
#11727=DIRECTION('center_axis',(5.97168109510217E-21,-1.,-1.13946463231163E-19));
#11728=DIRECTION('ref_axis',(0.688354575693753,0.,0.725374371012289));
#11729=DIRECTION('',(-5.97168109510217E-21,1.,1.13946463231163E-19));
#11730=DIRECTION('',(5.97168109510217E-21,-1.,-1.13946463231163E-19));
#11731=DIRECTION('center_axis',(0.998629534754574,0.,-0.0523359562429438));
#11732=DIRECTION('ref_axis',(-0.0523359562429438,0.,-0.998629534754574));
#11733=DIRECTION('center_axis',(4.10828654779316E-33,-1.13946463231163E-19,
1.));
#11734=DIRECTION('ref_axis',(1.,0.,-4.10828654779316E-33));
#11735=DIRECTION('center_axis',(-0.998629534754574,0.,-0.0523359562429455));
#11736=DIRECTION('ref_axis',(-0.0523359562429455,0.,0.998629534754574));
#14938=CARTESIAN_POINT('',(0.,0.,0.));
#14939=CARTESIAN_POINT('Origin',(8.1,-1.,0.7));
#14940=CARTESIAN_POINT('',(7.94916965151797,-1.19937453693185,0.7));
#14941=CARTESIAN_POINT('',(8.26514540988519,-1.18768855477586,0.7));
#14942=CARTESIAN_POINT('Ctrl Pts',(7.94916965151797,-1.19937453693185,0.7));
#14943=CARTESIAN_POINT('Ctrl Pts',(7.97160858810976,-1.21634998764782,0.7));
#14944=CARTESIAN_POINT('Ctrl Pts',(7.99739856866269,-1.22989011121344,0.69528529300377));
#14945=CARTESIAN_POINT('Ctrl Pts',(8.03944443766207,-1.24298414277179,0.688517705185315));
#14946=CARTESIAN_POINT('Ctrl Pts',(8.05362924383607,-1.24609346022897,0.686388676887586));
#14947=CARTESIAN_POINT('Ctrl Pts',(8.075506183533,-1.24890990228851,0.684139035126277));
#14948=CARTESIAN_POINT('Ctrl Pts',(8.08297567221474,-1.24953307703463,0.683546226354886));
#14949=CARTESIAN_POINT('Ctrl Pts',(8.0940066533036,-1.24995288972095,0.68299521602547));
#14950=CARTESIAN_POINT('Ctrl Pts',(8.09752287926269,-1.25001251279495,0.68286729538075));
#14951=CARTESIAN_POINT('Ctrl Pts',(8.10293413375911,-1.249989933108,0.682747340264197));
#14952=CARTESIAN_POINT('Ctrl Pts',(8.10482478940148,-1.24996059450444,0.682719828470948));
#14953=CARTESIAN_POINT('Ctrl Pts',(8.10828546792054,-1.24986760009171,0.682696100760705));
#14954=CARTESIAN_POINT('Ctrl Pts',(8.10985478687837,-1.24981062779486,0.682695370268813));
#14955=CARTESIAN_POINT('Ctrl Pts',(8.11326464342549,-1.24965465239671,0.682715595753076));
#14956=CARTESIAN_POINT('Ctrl Pts',(8.11510409202247,-1.2495501177419,0.682740330911594));
#14957=CARTESIAN_POINT('Ctrl Pts',(8.12014207260669,-1.24920790966494,0.682845651127781));
#14958=CARTESIAN_POINT('Ctrl Pts',(8.12333423895876,-1.24892926854386,0.682953992816581));
#14959=CARTESIAN_POINT('Ctrl Pts',(8.139194120874,-1.2472372768871,0.683691668462565));
#14960=CARTESIAN_POINT('Ctrl Pts',(8.15164141295685,-1.2449338270761,0.684918799511701));
#14961=CARTESIAN_POINT('Ctrl Pts',(8.19196937649467,-1.23428099896052,0.690212518998986));
#14962=CARTESIAN_POINT('Ctrl Pts',(8.21811504697062,-1.22213176592155,0.695755006185672));
#14963=CARTESIAN_POINT('Ctrl Pts',(8.24962874265135,-1.20052913769617,0.699397421419897));
#14964=CARTESIAN_POINT('Ctrl Pts',(8.25758631484639,-1.19433973204149,0.7));
#14965=CARTESIAN_POINT('Ctrl Pts',(8.26514540988519,-1.18768855477586,0.7));
#14966=CARTESIAN_POINT('Origin',(8.1,-1.,0.7));
#14967=CARTESIAN_POINT('Origin',(2.7,1.,0.7));
#14968=CARTESIAN_POINT('',(2.8076286513348,1.22564590451442,0.7));
#14969=CARTESIAN_POINT('',(2.57739843082973,1.21787348447435,0.7));
#14970=CARTESIAN_POINT('Ctrl Pts',(2.80762864495888,1.22564590575571,0.7));
#14971=CARTESIAN_POINT('Ctrl Pts',(2.78743249310418,1.23527907171202,0.7));
#14972=CARTESIAN_POINT('Ctrl Pts',(2.76507271635938,1.24261561512899,0.698430289974852));
#14973=CARTESIAN_POINT('Ctrl Pts',(2.73219941643314,1.24807722603274,0.696876198609429));
#14974=CARTESIAN_POINT('Ctrl Pts',(2.72335305886828,1.24906618730719,0.696525251810408));
#14975=CARTESIAN_POINT('Ctrl Pts',(2.71018695034311,1.24982905432238,0.696188910804419));
#14976=CARTESIAN_POINT('Ctrl Pts',(2.70590779780308,1.24996687586326,0.696107915309552));
#14977=CARTESIAN_POINT('Ctrl Pts',(2.69921702211412,1.25001037316246,0.696030339680738));
#14978=CARTESIAN_POINT('Ctrl Pts',(2.69680890442544,1.24999123464332,0.696012302673685));
#14979=CARTESIAN_POINT('Ctrl Pts',(2.69234597975348,1.24989125947742,0.695997601992606));
#14980=CARTESIAN_POINT('Ctrl Pts',(2.69029169500035,1.24981988388707,0.69599819279703));
#14981=CARTESIAN_POINT('Ctrl Pts',(2.6857660481318,1.24960673159635,0.696015705561832));
#14982=CARTESIAN_POINT('Ctrl Pts',(2.68329599580702,1.24945360531346,0.696035938105249));
#14983=CARTESIAN_POINT('Ctrl Pts',(2.67625328071593,1.24891193026541,0.696123377063474));
#14984=CARTESIAN_POINT('Ctrl Pts',(2.67169109188753,1.24843439216159,0.696216059649547));
#14985=CARTESIAN_POINT('Ctrl Pts',(2.64765560351845,1.24524789167778,0.696873729305584));
#14986=CARTESIAN_POINT('Ctrl Pts',(2.62857598726268,1.24037162800668,0.698048768812303));
#14987=CARTESIAN_POINT('Ctrl Pts',(2.59902076831046,1.22902239593109,0.699541037747764));
#14988=CARTESIAN_POINT('Ctrl Pts',(2.58799157881597,1.22383445108162,0.7));
#14989=CARTESIAN_POINT('Ctrl Pts',(2.57739843082979,1.21787348447436,0.7));
#14990=CARTESIAN_POINT('Origin',(2.7,1.,0.7));
#14991=CARTESIAN_POINT('Origin',(2.7,-1.,0.7));
#14992=CARTESIAN_POINT('',(2.57739843082979,-1.21787348447436,0.7));
#14993=CARTESIAN_POINT('',(2.80762864495888,-1.22564590575571,0.7));
#14994=CARTESIAN_POINT('Ctrl Pts',(2.57739843082979,-1.21787348447436,0.7));
#14995=CARTESIAN_POINT('Ctrl Pts',(2.59689796709118,-1.22884624579732,0.7));
#14996=CARTESIAN_POINT('Ctrl Pts',(2.61871070177046,-1.23767364961455,0.698430520021629));
#14997=CARTESIAN_POINT('Ctrl Pts',(2.6511387549791,-1.24533993869645,0.696876447160353));
#14998=CARTESIAN_POINT('Ctrl Pts',(2.65989793055836,-1.24692336726652,0.696525471319567));
#14999=CARTESIAN_POINT('Ctrl Pts',(2.67298219502323,-1.24857266139659,0.696189053183015));
#15000=CARTESIAN_POINT('Ctrl Pts',(2.67724223626036,-1.24899884484677,0.696108027479433));
#15001=CARTESIAN_POINT('Ctrl Pts',(2.68391475503581,-1.24949361628703,0.696030400846995));
#15002=CARTESIAN_POINT('Ctrl Pts',(2.68631866330158,-1.24963697932539,0.69601234479389));
#15003=CARTESIAN_POINT('Ctrl Pts',(2.69077815115796,-1.24983831390468,0.695997608323079));
#15004=CARTESIAN_POINT('Ctrl Pts',(2.69283257145917,-1.24990568929416,0.695998182544699));
#15005=CARTESIAN_POINT('Ctrl Pts',(2.69736230434386,-1.24999833696454,0.696015659042177));
#15006=CARTESIAN_POINT('Ctrl Pts',(2.69983707579759,-1.25001219669429,0.696035872086962));
#15007=CARTESIAN_POINT('Ctrl Pts',(2.70690037992806,-1.24994687665095,0.696123257636812));
#15008=CARTESIAN_POINT('Ctrl Pts',(2.71148446565418,-1.24977820005943,0.696215908504701));
#15009=CARTESIAN_POINT('Ctrl Pts',(2.73568105999059,-1.24822038288304,0.696873447340259));
#15010=CARTESIAN_POINT('Ctrl Pts',(2.75504695022812,-1.24464213141243,0.698048515307351));
#15011=CARTESIAN_POINT('Ctrl Pts',(2.78530198112344,-1.2353118289445,0.699540950501024));
#15012=CARTESIAN_POINT('Ctrl Pts',(2.79665680001786,-1.23087925931356,0.7));
#15013=CARTESIAN_POINT('Ctrl Pts',(2.80762864495888,-1.22564590575571,0.7));
#15014=CARTESIAN_POINT('Origin',(2.7,-1.,0.7));
#15015=CARTESIAN_POINT('Origin',(8.1,1.,0.7));
#15016=CARTESIAN_POINT('',(8.26514540988519,1.18768855477586,0.7));
#15017=CARTESIAN_POINT('',(7.94916965249954,1.19937453719419,0.7));
#15018=CARTESIAN_POINT('Ctrl Pts',(8.26514540988519,1.18768855477586,0.7));
#15019=CARTESIAN_POINT('Ctrl Pts',(8.24402114884725,1.20627559516199,0.7));
#15020=CARTESIAN_POINT('Ctrl Pts',(8.21930102059268,1.22168408824046,0.695284768760077));
#15021=CARTESIAN_POINT('Ctrl Pts',(8.17833936508797,1.23784683595578,0.688517484674842));
#15022=CARTESIAN_POINT('Ctrl Pts',(8.16442627443898,1.24199461640617,0.686388979601913));
#15023=CARTESIAN_POINT('Ctrl Pts',(8.14282164862934,1.24641910835203,0.684139556285851));
#15024=CARTESIAN_POINT('Ctrl Pts',(8.13541969045672,1.24759243465272,0.683546718614312));
#15025=CARTESIAN_POINT('Ctrl Pts',(8.12445132655127,1.24882623938238,0.682995554842566));
#15026=CARTESIAN_POINT('Ctrl Pts',(8.12094947916695,1.24914555886372,0.68286756899844));
#15027=CARTESIAN_POINT('Ctrl Pts',(8.11555178799172,1.24952297970176,0.682747494033431));
#15028=CARTESIAN_POINT('Ctrl Pts',(8.11366421100955,1.24963346420394,0.682719937279798));
#15029=CARTESIAN_POINT('Ctrl Pts',(8.11020620287515,1.24979651712922,0.682696124556263));
#15030=CARTESIAN_POINT('Ctrl Pts',(8.10863696767328,1.24985569708818,0.682695355189016));
#15031=CARTESIAN_POINT('Ctrl Pts',(8.10522484403353,1.249952190393,0.682715496638402));
#15032=CARTESIAN_POINT('Ctrl Pts',(8.10338263267786,1.24998390529834,0.682740187713169));
#15033=CARTESIAN_POINT('Ctrl Pts',(8.09833277498968,1.25001501472208,0.682845394223802));
#15034=CARTESIAN_POINT('Ctrl Pts',(8.09512844909059,1.24997307323179,0.682953673497893));
#15035=CARTESIAN_POINT('Ctrl Pts',(8.07918314804204,1.24945780552822,0.683691186949858));
#15036=CARTESIAN_POINT('Ctrl Pts',(8.06659630270856,1.24808001426183,0.684918585227095));
#15037=CARTESIAN_POINT('Ctrl Pts',(8.02558960427868,1.24043495378573,0.69021260546313));
#15038=CARTESIAN_POINT('Ctrl Pts',(7.9986188553413,1.2302509517108,0.695754623970086));
#15039=CARTESIAN_POINT('Ctrl Pts',(7.96559475436581,1.21103543221342,0.69939729083119));
#15040=CARTESIAN_POINT('Ctrl Pts',(7.95720051358587,1.20545002552208,0.7));
#15041=CARTESIAN_POINT('Ctrl Pts',(7.94916965151797,1.19937453693185,0.7));
#15042=CARTESIAN_POINT('Origin',(8.1,1.,0.7));
#15043=CARTESIAN_POINT('Ctrl Pts',(1.1,1.14549341399196,0.7));
#15044=CARTESIAN_POINT('Ctrl Pts',(1.89984199608574,1.1957170361627,0.7));
#15045=CARTESIAN_POINT('Ctrl Pts',(2.70080437300401,1.2273695200909,0.7));
#15046=CARTESIAN_POINT('Ctrl Pts',(3.50204003610941,1.24374118183538,0.7));
#15047=CARTESIAN_POINT('Ctrl Pts',(1.09819048660397,1.17431102498992,0.7));
#15048=CARTESIAN_POINT('Ctrl Pts',(1.89847848223077,1.22458382597074,0.70000077422621));
#15049=CARTESIAN_POINT('Ctrl Pts',(2.69984520196781,1.25626413437997,0.699999727319846));
#15050=CARTESIAN_POINT('Ctrl Pts',(3.50144932661635,1.27265074030048,0.700000000000001));
#15051=CARTESIAN_POINT('Ctrl Pts',(1.09505363188407,1.22426736091617,0.676703190608825));
#15052=CARTESIAN_POINT('Ctrl Pts',(1.89610976425884,1.27462253270773,0.67666760713801));
#15053=CARTESIAN_POINT('Ctrl Pts',(2.69818680938115,1.3063522351595,0.67664530655333));
#15054=CARTESIAN_POINT('Ctrl Pts',(3.50042536655637,1.322763754511,0.676632802377821));
#15055=CARTESIAN_POINT('Ctrl Pts',(1.09381704710221,1.24396073223232,0.627109609335854));
#15056=CARTESIAN_POINT('Ctrl Pts',(1.89518106151152,1.29430885982199,0.62701751976321));
#15057=CARTESIAN_POINT('Ctrl Pts',(2.69753328610131,1.32603127467068,0.626959208652505));
#15058=CARTESIAN_POINT('Ctrl Pts',(3.50002334924346,1.34243864233338,0.626926882269943));
#15059=CARTESIAN_POINT('Ctrl Pts',(1.09374258853658,1.24514653057163,0.605486452199395));
#15060=CARTESIAN_POINT('Ctrl Pts',(1.89512529323683,1.29547288309274,0.605377720397184));
#15061=CARTESIAN_POINT('Ctrl Pts',(2.69749615303001,1.32718177535833,0.605308474776761));
#15062=CARTESIAN_POINT('Ctrl Pts',(3.5,1.34358136363184,0.605270327458635));
#15063=CARTESIAN_POINT('',(1.1,1.14549341399195,0.7));
#15064=CARTESIAN_POINT('Ctrl Pts',(1.1,1.14549341399196,0.7));
#15065=CARTESIAN_POINT('Ctrl Pts',(1.59210562457523,1.17639367564078,0.7));
#15066=CARTESIAN_POINT('Ctrl Pts',(2.08463535466703,1.20026407570248,0.7));
#15067=CARTESIAN_POINT('Ctrl Pts',(2.57739190516306,1.2178709162388,0.7));
#15068=CARTESIAN_POINT('',(1.1,1.24553911298206,0.605485603995113));
#15069=CARTESIAN_POINT('Ctrl Pts',(1.1,1.14549341399196,0.7));
#15070=CARTESIAN_POINT('Ctrl Pts',(1.1,1.15341616150799,0.7));
#15071=CARTESIAN_POINT('Ctrl Pts',(1.1000012416168,1.16127613060545,0.699006361583129));
#15072=CARTESIAN_POINT('Ctrl Pts',(1.10000231308998,1.16893252943985,0.697119293189023));
#15073=CARTESIAN_POINT('Ctrl Pts',(1.10000291357081,1.17322337016277,0.696061732044743));
#15074=CARTESIAN_POINT('Ctrl Pts',(1.10000345673767,1.17745032641463,0.694722535963768));
#15075=CARTESIAN_POINT('Ctrl Pts',(1.10000379529503,1.18158693416151,0.693112479763539));
#15076=CARTESIAN_POINT('Ctrl Pts',(1.1000044034764,1.18901789868739,0.690220189452084));
#15077=CARTESIAN_POINT('Ctrl Pts',(1.1000042334852,1.19607766167095,0.686488065947256));
#15078=CARTESIAN_POINT('Ctrl Pts',(1.10000339376692,1.2026196529327,0.681996646156542));
#15079=CARTESIAN_POINT('Ctrl Pts',(1.10000293249552,1.20621327895058,0.67952943359521));
#15080=CARTESIAN_POINT('Ctrl Pts',(1.10000228571683,1.20965039763183,0.676832226278619));
#15081=CARTESIAN_POINT('Ctrl Pts',(1.10000171524363,1.21290279159005,0.673912896410569));
#15082=CARTESIAN_POINT('Ctrl Pts',(1.10000115816795,1.2160788033717,0.671062126739188));
#15083=CARTESIAN_POINT('Ctrl Pts',(1.10000066850715,1.2190594221245,0.668016750164662));
#15084=CARTESIAN_POINT('Ctrl Pts',(1.10000067525152,1.22182202639256,0.664788091882127));
#15085=CARTESIAN_POINT('Ctrl Pts',(1.10000068775799,1.22694487635592,0.658801012170571));
#15086=CARTESIAN_POINT('Ctrl Pts',(1.10000222199399,1.23132099043293,0.652185071179834));
#15087=CARTESIAN_POINT('Ctrl Pts',(1.10000276904041,1.23488987417606,0.64510534613808));
#15088=CARTESIAN_POINT('Ctrl Pts',(1.10000282439334,1.23525099193115,0.644388983656765));
#15089=CARTESIAN_POINT('Ctrl Pts',(1.10000287212626,1.23560380546488,0.64366785367332));
#15090=CARTESIAN_POINT('Ctrl Pts',(1.10000291138002,1.23594822450451,0.642942116631622));
#15091=CARTESIAN_POINT('Ctrl Pts',(1.10000329911404,1.23935026814133,0.635773555081239));
#15092=CARTESIAN_POINT('Ctrl Pts',(1.10000258010782,1.24189771450306,0.628240464257889));
#15093=CARTESIAN_POINT('Ctrl Pts',(1.10000149084855,1.24353681278199,0.620511076118615));
#15094=CARTESIAN_POINT('Ctrl Pts',(1.10000079446814,1.24458471384188,0.615569557890241));
#15095=CARTESIAN_POINT('Ctrl Pts',(1.10000000111128,1.24526049271905,0.610547146027233));
#15096=CARTESIAN_POINT('Ctrl Pts',(1.09999999916631,1.24553911263843,0.605485603997432));
#15097=CARTESIAN_POINT('',(3.5,1.34358136363184,0.605270327458635));
#15098=CARTESIAN_POINT('Ctrl Pts',(3.5,1.34358136363184,0.605270327458635));
#15099=CARTESIAN_POINT('Ctrl Pts',(2.6995848679345,1.32722445934619,0.605308375488923));
#15100=CARTESIAN_POINT('Ctrl Pts',(1.89930203168261,1.29563783986497,0.605377360150118));
#15101=CARTESIAN_POINT('Ctrl Pts',(1.09999999916631,1.24553911263843,0.605485603997431));
#15102=CARTESIAN_POINT('',(3.5,1.24369946473792,0.7));
#15103=CARTESIAN_POINT('Ctrl Pts',(3.5,1.34358136363184,0.605270327458635));
#15104=CARTESIAN_POINT('Ctrl Pts',(3.5,1.34316359984937,0.613184373088104));
#15105=CARTESIAN_POINT('Ctrl Pts',(3.50000057901142,1.34177887744868,0.621008021569537));
#15106=CARTESIAN_POINT('Ctrl Pts',(3.50000082863025,1.33951086762262,0.628580534231506));
#15107=CARTESIAN_POINT('Ctrl Pts',(3.50000096811,1.33824356956914,0.632811834486987));
#15108=CARTESIAN_POINT('Ctrl Pts',(3.50000102536574,1.33669948631919,0.636964759527324));
#15109=CARTESIAN_POINT('Ctrl Pts',(3.50000098105742,1.334886463945,0.641009258704104));
#15110=CARTESIAN_POINT('Ctrl Pts',(3.50000090179773,1.3316432906201,0.648244145614236));
#15111=CARTESIAN_POINT('Ctrl Pts',(3.50000044940971,1.3275777080273,0.655054131048541));
#15112=CARTESIAN_POINT('Ctrl Pts',(3.50000027423476,1.32275302640998,0.661275670751788));
#15113=CARTESIAN_POINT('Ctrl Pts',(3.50000024156065,1.32185311357394,0.66243612938574));
#15114=CARTESIAN_POINT('Ctrl Pts',(3.50000022115524,1.32092666334894,0.663576045687695));
#15115=CARTESIAN_POINT('Ctrl Pts',(3.50000022069074,1.31997391848392,0.664694242102532));
#15116=CARTESIAN_POINT('Ctrl Pts',(3.50000021976176,1.31806844339147,0.666930617752677));
#15117=CARTESIAN_POINT('Ctrl Pts',(3.50000029790302,1.31605782519,0.669080165434128));
#15118=CARTESIAN_POINT('Ctrl Pts',(3.50000040488465,1.31394946763378,0.671139079687271));
#15119=CARTESIAN_POINT('Ctrl Pts',(3.50000069329649,1.3082655455861,0.6766897075128));
#15120=CARTESIAN_POINT('Ctrl Pts',(3.5000011432336,1.30193818666762,0.681521899278667));
#15121=CARTESIAN_POINT('Ctrl Pts',(3.50000129797765,1.29513115062548,0.68558123547136));
#15122=CARTESIAN_POINT('Ctrl Pts',(3.50000139624096,1.2908086457691,0.688158936000333));
#15123=CARTESIAN_POINT('Ctrl Pts',(3.50000139493488,1.28629176508013,0.690424313967808));
#15124=CARTESIAN_POINT('Ctrl Pts',(3.50000129141552,1.28161680488022,0.692354162840695));
#15125=CARTESIAN_POINT('Ctrl Pts',(3.50000112941005,1.27430059661786,0.695374333209024));
#15126=CARTESIAN_POINT('Ctrl Pts',(3.5000007162179,1.26668229982361,0.697540280949125));
#15127=CARTESIAN_POINT('Ctrl Pts',(3.50000038344698,1.25890895215876,0.698782355543395));
#15128=CARTESIAN_POINT('Ctrl Pts',(3.50000016866387,1.25389173534334,0.699584038140014));
#15129=CARTESIAN_POINT('Ctrl Pts',(3.4999999993056,1.24880933504677,0.69999999987784));
#15130=CARTESIAN_POINT('Ctrl Pts',(3.49999999991873,1.24369946470729,0.7));
#15131=CARTESIAN_POINT('Ctrl Pts',(2.80762377174497,1.22564400643366,0.7));
#15132=CARTESIAN_POINT('Ctrl Pts',(3.03837960601223,1.23298334400942,0.7));
#15133=CARTESIAN_POINT('Ctrl Pts',(3.26917843294065,1.23897560812206,0.7));
#15134=CARTESIAN_POINT('Ctrl Pts',(3.49999999991873,1.24369946470729,0.7));
#15135=CARTESIAN_POINT('Ctrl Pts',(7.29709043526678,1.22049830417059,0.7));
#15136=CARTESIAN_POINT('Ctrl Pts',(8.19846709497879,1.19422430779862,0.7));
#15137=CARTESIAN_POINT('Ctrl Pts',(9.09944331332256,1.15544418981837,0.7));
#15138=CARTESIAN_POINT('Ctrl Pts',(10.,1.10900986674273,0.7));
#15139=CARTESIAN_POINT('Ctrl Pts',(7.29793284700474,1.24939875264889,0.7));
#15140=CARTESIAN_POINT('Ctrl Pts',(8.19957769811722,1.22310890030201,0.699999704549177));
#15141=CARTESIAN_POINT('Ctrl Pts',(9.10076698492607,1.18430758604571,0.700000491839571));
#15142=CARTESIAN_POINT('Ctrl Pts',(10.0014871213396,1.13785139984992,0.7));
#15143=CARTESIAN_POINT('Ctrl Pts',(7.29939288958794,1.29948813715084,0.676630595533454));
#15144=CARTESIAN_POINT('Ctrl Pts',(8.20149954052228,1.27317186922949,0.676644146017132));
#15145=CARTESIAN_POINT('Ctrl Pts',(9.10306300621911,1.23433322993607,0.676664155483857));
#15146=CARTESIAN_POINT('Ctrl Pts',(10.0040646682326,1.18784086746588,0.676686753673613));
#15147=CARTESIAN_POINT('Ctrl Pts',(7.29996660609513,1.31917051289423,0.626939603849942));
#15148=CARTESIAN_POINT('Ctrl Pts',(8.20225661204673,1.29285896783792,0.626974637782525));
#15149=CARTESIAN_POINT('Ctrl Pts',(9.10396596140606,1.25402923300358,0.627026849623412));
#15150=CARTESIAN_POINT('Ctrl Pts',(10.0050807923581,1.20754778500352,0.627085325222079));
#15151=CARTESIAN_POINT('Ctrl Pts',(7.29999999953093,1.32031613471704,0.605285370449856));
#15152=CARTESIAN_POINT('Ctrl Pts',(8.20230020786565,1.29401302889245,0.605326714446839));
#15153=CARTESIAN_POINT('Ctrl Pts',(9.10401978846669,1.25519559703033,0.605388684776982));
#15154=CARTESIAN_POINT('Ctrl Pts',(10.0051416645797,1.20872835322339,0.605457722909465));
#15155=CARTESIAN_POINT('',(7.29999999989017,1.22041345054104,0.7));
#15156=CARTESIAN_POINT('Ctrl Pts',(7.29999999978094,1.22041345055303,0.7));
#15157=CARTESIAN_POINT('Ctrl Pts',(7.51641201913776,1.21409884615949,0.7));
#15158=CARTESIAN_POINT('Ctrl Pts',(7.73280095443524,1.20706364503479,0.7));
#15159=CARTESIAN_POINT('Ctrl Pts',(7.94916654146952,1.19937499621344,0.7));
#15160=CARTESIAN_POINT('',(7.29999999953133,1.3203161347307,0.605285370449834));
#15161=CARTESIAN_POINT('Ctrl Pts',(7.29999999989087,1.22041345054982,0.7));
#15162=CARTESIAN_POINT('Ctrl Pts',(7.30000000079355,1.22832360919786,0.699999999740221));
#15163=CARTESIAN_POINT('Ctrl Pts',(7.29999941101664,1.23617007614594,0.699006006469939));
#15164=CARTESIAN_POINT('Ctrl Pts',(7.29999889581476,1.24381267896118,0.697118889344366));
#15165=CARTESIAN_POINT('Ctrl Pts',(7.29999860583198,1.24811433880851,0.696056720321257));
#15166=CARTESIAN_POINT('Ctrl Pts',(7.29999834128398,1.25235147078274,0.694710570513598));
#15167=CARTESIAN_POINT('Ctrl Pts',(7.29999817264931,1.25649739217805,0.693091458416622));
#15168=CARTESIAN_POINT('Ctrl Pts',(7.29999787070862,1.26392067210813,0.690192435210923));
#15169=CARTESIAN_POINT('Ctrl Pts',(7.29999793286912,1.27097116792553,0.686452948287278));
#15170=CARTESIAN_POINT('Ctrl Pts',(7.2999983123982,1.27750284616821,0.681954753865011));
#15171=CARTESIAN_POINT('Ctrl Pts',(7.2999985213788,1.28109939299731,0.679477906983553));
#15172=CARTESIAN_POINT('Ctrl Pts',(7.29999881895966,1.28453837241868,0.676770138671336));
#15173=CARTESIAN_POINT('Ctrl Pts',(7.29999908362886,1.28779148632494,0.673839551409954));
#15174=CARTESIAN_POINT('Ctrl Pts',(7.29999934163235,1.29096267037196,0.670982771155867));
#15175=CARTESIAN_POINT('Ctrl Pts',(7.29999957112158,1.2939379836903,0.667931525418885));
#15176=CARTESIAN_POINT('Ctrl Pts',(7.29999957127586,1.29669488996436,0.664697318929259));
#15177=CARTESIAN_POINT('Ctrl Pts',(7.29999957156178,1.30180432468448,0.658703293276094));
#15178=CARTESIAN_POINT('Ctrl Pts',(7.29999886995656,1.30616650855536,0.652082235935803));
#15179=CARTESIAN_POINT('Ctrl Pts',(7.29999863193158,1.30972187224872,0.644999691185358));
#15180=CARTESIAN_POINT('Ctrl Pts',(7.29999860759325,1.31008541227461,0.644275492840527));
#15181=CARTESIAN_POINT('Ctrl Pts',(7.29999858692673,1.31044047656777,0.643546449710686));
#15182=CARTESIAN_POINT('Ctrl Pts',(7.29999857034625,1.31078697300061,0.642812727646596));
#15183=CARTESIAN_POINT('Ctrl Pts',(7.29999840819729,1.31417553742296,0.635637287305567));
#15184=CARTESIAN_POINT('Ctrl Pts',(7.29999876577208,1.31670951795567,0.628098908385918));
#15185=CARTESIAN_POINT('Ctrl Pts',(7.29999928780719,1.3183355664444,0.620365998324013));
#15186=CARTESIAN_POINT('Ctrl Pts',(7.29999962266353,1.3193785856694,0.615405768714856));
#15187=CARTESIAN_POINT('Ctrl Pts',(7.3,1.32004717656055,0.610364828659741));
#15188=CARTESIAN_POINT('Ctrl Pts',(7.3,1.32031613470337,0.605285370449877));
#15189=CARTESIAN_POINT('',(10.,1.20899340483173,0.605457329065657));
#15190=CARTESIAN_POINT('Ctrl Pts',(9.99999999968202,1.20899340489109,0.605457329065633));
#15191=CARTESIAN_POINT('Ctrl Pts',(9.10058974048747,1.25534320916473,0.605388449123016));
#15192=CARTESIAN_POINT('Ctrl Pts',(8.20058408060299,1.29406305600824,0.605326635812744));
#15193=CARTESIAN_POINT('Ctrl Pts',(7.29999999953093,1.32031613471704,0.605285370449856));
#15194=CARTESIAN_POINT('',(9.99999999523418,1.1090098672342,0.7));
#15195=CARTESIAN_POINT('Ctrl Pts',(9.99999999968202,1.20899340489109,0.605457329065633));
#15196=CARTESIAN_POINT('Ctrl Pts',(9.99999999887489,1.20856043137698,0.613368813757176));
#15197=CARTESIAN_POINT('Ctrl Pts',(9.99999852309337,1.20715974444566,0.621187403383205));
#15198=CARTESIAN_POINT('Ctrl Pts',(9.99999786661901,1.20487567413208,0.628752957409046));
#15199=CARTESIAN_POINT('Ctrl Pts',(9.9999975031266,1.20361097553651,0.63294203403));
#15200=CARTESIAN_POINT('Ctrl Pts',(9.99999733971606,1.20207445367248,0.63705356322819));
#15201=CARTESIAN_POINT('Ctrl Pts',(9.99999742766416,1.20027388348257,0.64105842070465));
#15202=CARTESIAN_POINT('Ctrl Pts',(9.9999975865154,1.19702170610966,0.6482919664668));
#15203=CARTESIAN_POINT('Ctrl Pts',(9.99999868569093,1.19294650045069,0.655099368158521));
#15204=CARTESIAN_POINT('Ctrl Pts',(9.9999991134218,1.18811276085989,0.661317774786376));
#15205=CARTESIAN_POINT('Ctrl Pts',(9.99999919410111,1.18720101282252,0.662490701033652));
#15206=CARTESIAN_POINT('Ctrl Pts',(9.99999924414009,1.18626214680169,0.663642601192937));
#15207=CARTESIAN_POINT('Ctrl Pts',(9.99999924372355,1.18529642131707,0.664772262763739));
#15208=CARTESIAN_POINT('Ctrl Pts',(9.99999924291654,1.18342543943696,0.666960851926287));
#15209=CARTESIAN_POINT('Ctrl Pts',(9.99999905429896,1.18145367213587,0.669066014649603));
#15210=CARTESIAN_POINT('Ctrl Pts',(9.99999879621773,1.17938809187152,0.671084194359814));
#15211=CARTESIAN_POINT('Ctrl Pts',(9.99999808597787,1.17370361260899,0.676638227242868));
#15212=CARTESIAN_POINT('Ctrl Pts',(9.9999969699445,1.16737553754052,0.681473799108647));
#15213=CARTESIAN_POINT('Ctrl Pts',(9.99999660204079,1.16056788011185,0.685537070165577));
#15214=CARTESIAN_POINT('Ctrl Pts',(9.99999636768906,1.15623145667386,0.688125341392612));
#15215=CARTESIAN_POINT('Ctrl Pts',(9.99999638726733,1.15169947441128,0.690399565850749));
#15216=CARTESIAN_POINT('Ctrl Pts',(9.99999666360534,1.14700857532255,0.692336497939236));
#15217=CARTESIAN_POINT('Ctrl Pts',(9.99999709503399,1.13968497812548,0.695360504669253));
#15218=CARTESIAN_POINT('Ctrl Pts',(9.99999815490668,1.13205884654683,0.697530003145419));
#15219=CARTESIAN_POINT('Ctrl Pts',(9.99999900983214,1.12427739544825,0.698775573347137));
#15220=CARTESIAN_POINT('Ctrl Pts',(9.99999956314479,1.11924119569193,0.699581713521624));
#15221=CARTESIAN_POINT('Ctrl Pts',(10.,1.11413933950174,0.7));
#15222=CARTESIAN_POINT('Ctrl Pts',(10.,1.10900986674273,0.7));
#15223=CARTESIAN_POINT('Ctrl Pts',(8.26514054272776,1.18768929227839,0.7));
#15224=CARTESIAN_POINT('Ctrl Pts',(8.84359655063997,1.16547286645366,0.7));
#15225=CARTESIAN_POINT('Ctrl Pts',(9.42188471826001,1.13881853081542,0.7));
#15226=CARTESIAN_POINT('Ctrl Pts',(9.99999999522154,1.10900986698912,0.7));
#15227=CARTESIAN_POINT('Origin',(5.4,-8.11656130105013E-18,0.7));
#15228=CARTESIAN_POINT('',(7.3,-1.22041345053557,0.7));
#15229=CARTESIAN_POINT('Ctrl Pts',(7.94916654049851,-1.19937499624794,0.7));
#15230=CARTESIAN_POINT('Ctrl Pts',(7.73280095382446,-1.20706364505454,0.7));
#15231=CARTESIAN_POINT('Ctrl Pts',(7.51641201888728,-1.21409884616656,0.7));
#15232=CARTESIAN_POINT('Ctrl Pts',(7.29999999989085,-1.22041345054982,0.7));
#15233=CARTESIAN_POINT('',(7.3,-0.712777777777778,0.7));
#15234=CARTESIAN_POINT('',(10.,-1.10900986674244,0.7));
#15235=CARTESIAN_POINT('',(10.,0.653773457742722,0.7));
#15236=CARTESIAN_POINT('Ctrl Pts',(10.,-1.10900986674273,0.7));
#15237=CARTESIAN_POINT('Ctrl Pts',(9.42188472144661,-1.13881853066854,0.7));
#15238=CARTESIAN_POINT('Ctrl Pts',(8.84359655223373,-1.16547286639245,0.7));
#15239=CARTESIAN_POINT('Ctrl Pts',(8.26514054272776,-1.18768929227839,0.7));
#15240=CARTESIAN_POINT('',(7.95,-1.,0.7));
#15241=CARTESIAN_POINT('Origin',(8.1,-1.,0.7));
#15242=CARTESIAN_POINT('',(7.95,1.,0.7));
#15243=CARTESIAN_POINT('Origin',(8.1,1.,0.7));
#15244=CARTESIAN_POINT('',(8.4,-4.89858719658942E-17,0.7));
#15245=CARTESIAN_POINT('Origin',(8.8,0.,0.7));
#15246=CARTESIAN_POINT('Origin',(8.1,-1.,0.8));
#15247=CARTESIAN_POINT('',(7.95,-1.,0.9));
#15248=CARTESIAN_POINT('Origin',(8.1,-1.,0.9));
#15249=CARTESIAN_POINT('',(7.95,-1.,0.8));
#15250=CARTESIAN_POINT('Origin',(2.7,-1.,0.8));
#15251=CARTESIAN_POINT('',(2.55,-1.,0.9));
#15252=CARTESIAN_POINT('Origin',(2.7,-1.,0.9));
#15253=CARTESIAN_POINT('',(2.55,-1.,0.7));
#15254=CARTESIAN_POINT('',(2.55,-1.,0.8));
#15255=CARTESIAN_POINT('Origin',(2.7,-1.,0.7));
#15256=CARTESIAN_POINT('Origin',(2.7,1.,0.8));
#15257=CARTESIAN_POINT('',(2.55,1.,0.9));
#15258=CARTESIAN_POINT('Origin',(2.7,1.,0.9));
#15259=CARTESIAN_POINT('',(2.55,1.,0.7));
#15260=CARTESIAN_POINT('',(2.55,1.,0.8));
#15261=CARTESIAN_POINT('Origin',(2.7,1.,0.7));
#15262=CARTESIAN_POINT('Origin',(8.1,1.,0.8));
#15263=CARTESIAN_POINT('',(7.95,1.,0.9));
#15264=CARTESIAN_POINT('Origin',(8.1,1.,0.9));
#15265=CARTESIAN_POINT('',(7.95,1.,0.8));
#15266=CARTESIAN_POINT('Origin',(2.,0.,0.75));
#15267=CARTESIAN_POINT('',(1.7,3.67394039744206E-17,0.9));
#15268=CARTESIAN_POINT('Origin',(2.,0.,0.9));
#15269=CARTESIAN_POINT('',(1.7,3.67394039744206E-17,0.6));
#15270=CARTESIAN_POINT('',(1.7,3.67394039744206E-17,0.75));
#15271=CARTESIAN_POINT('Origin',(2.,0.,0.6));
#15272=CARTESIAN_POINT('Origin',(2.,0.,0.6));
#15273=CARTESIAN_POINT('',(1.83,-2.0818995585505E-17,0.6));
#15274=CARTESIAN_POINT('Origin',(2.,0.,0.6));
#15275=CARTESIAN_POINT('Origin',(8.8,0.,0.75));
#15276=CARTESIAN_POINT('',(8.5,3.67394039744206E-17,0.9));
#15277=CARTESIAN_POINT('Origin',(8.8,0.,0.9));
#15278=CARTESIAN_POINT('',(8.5,3.67394039744206E-17,0.6));
#15279=CARTESIAN_POINT('',(8.5,3.67394039744206E-17,0.75));
#15280=CARTESIAN_POINT('Origin',(8.8,0.,0.6));
#15281=CARTESIAN_POINT('Origin',(8.8,0.,0.6));
#15282=CARTESIAN_POINT('',(8.63,-2.0818995585505E-17,0.6));
#15283=CARTESIAN_POINT('Origin',(8.8,0.,0.6));
#15284=CARTESIAN_POINT('Origin',(2.,0.,0.45));
#15285=CARTESIAN_POINT('',(1.83,-2.0818995585505E-17,0.32));
#15286=CARTESIAN_POINT('',(1.83,2.0818995585505E-17,0.45));
#15287=CARTESIAN_POINT('Origin',(2.,0.,0.32));
#15288=CARTESIAN_POINT('Origin',(8.8,0.,0.45));
#15289=CARTESIAN_POINT('',(8.63,-2.0818995585505E-17,0.32));
#15290=CARTESIAN_POINT('',(8.63,2.0818995585505E-17,0.45));
#15291=CARTESIAN_POINT('Origin',(8.8,0.,0.32));
#15292=CARTESIAN_POINT('Origin',(10.,-0.62,0.32));
#15293=CARTESIAN_POINT('',(0.200274469199584,-0.62,0.));
#15294=CARTESIAN_POINT('',(0.217044958570157,-0.62,0.32));
#15295=CARTESIAN_POINT('',(0.221783445591644,-0.62,0.410415718550007));
#15296=CARTESIAN_POINT('',(0.,-0.62,0.));
#15297=CARTESIAN_POINT('',(7.7,-0.62,0.));
#15298=CARTESIAN_POINT('',(0.0167704893705732,-0.62,0.32));
#15299=CARTESIAN_POINT('',(0.0220575386407278,-0.62,0.420882909798596));
#15300=CARTESIAN_POINT('',(-0.1,-0.62,0.32));
#15301=CARTESIAN_POINT('Origin',(10.,-0.62,0.32));
#15302=CARTESIAN_POINT('',(0.9,-0.62,0.32));
#15303=CARTESIAN_POINT('',(0.9,-0.62,0.));
#15304=CARTESIAN_POINT('',(0.9,-0.62,0.16));
#15305=CARTESIAN_POINT('',(1.1,-0.62,0.32));
#15306=CARTESIAN_POINT('',(-0.1,-0.62,0.32));
#15307=CARTESIAN_POINT('',(1.1,-0.62,0.));
#15308=CARTESIAN_POINT('',(1.1,-0.62,0.16));
#15309=CARTESIAN_POINT('',(7.7,-0.62,0.));
#15310=CARTESIAN_POINT('Origin',(10.,-0.62,0.32));
#15311=CARTESIAN_POINT('',(3.5,-0.62,0.32));
#15312=CARTESIAN_POINT('',(3.5,-0.62,0.));
#15313=CARTESIAN_POINT('',(3.5,-0.62,0.16));
#15314=CARTESIAN_POINT('',(3.7,-0.62,0.32));
#15315=CARTESIAN_POINT('',(-0.1,-0.62,0.32));
#15316=CARTESIAN_POINT('',(3.7,-0.62,0.));
#15317=CARTESIAN_POINT('',(3.7,-0.62,0.16));
#15318=CARTESIAN_POINT('',(7.7,-0.62,0.));
#15319=CARTESIAN_POINT('Origin',(10.,-0.62,0.32));
#15320=CARTESIAN_POINT('',(7.1,-0.62,0.32));
#15321=CARTESIAN_POINT('',(7.1,-0.62,0.));
#15322=CARTESIAN_POINT('',(7.1,-0.62,0.16));
#15323=CARTESIAN_POINT('',(7.3,-0.62,0.32));
#15324=CARTESIAN_POINT('',(-0.1,-0.62,0.32));
#15325=CARTESIAN_POINT('',(7.3,-0.62,0.));
#15326=CARTESIAN_POINT('',(7.3,-0.62,0.16));
#15327=CARTESIAN_POINT('',(7.7,-0.62,0.));
#15328=CARTESIAN_POINT('Origin',(-0.0999999999999996,0.62,0.32));
#15329=CARTESIAN_POINT('',(0.217044958570158,0.62,0.32));
#15330=CARTESIAN_POINT('',(0.200274469199584,0.62,0.));
#15331=CARTESIAN_POINT('',(0.207951231396534,0.62,0.146481348799182));
#15332=CARTESIAN_POINT('',(0.0167704893705736,0.62,0.32));
#15333=CARTESIAN_POINT('',(10.,0.62,0.32));
#15334=CARTESIAN_POINT('',(0.,0.62,0.));
#15335=CARTESIAN_POINT('',(0.00822532444561912,0.62,0.156948540047771));
#15336=CARTESIAN_POINT('',(2.65,0.62,0.));
#15337=CARTESIAN_POINT('Origin',(-0.0999999999999996,0.62,0.32));
#15338=CARTESIAN_POINT('',(0.9,0.62,0.));
#15339=CARTESIAN_POINT('',(0.9,0.62,0.32));
#15340=CARTESIAN_POINT('',(0.9,0.62,0.16));
#15341=CARTESIAN_POINT('',(1.1,0.62,0.));
#15342=CARTESIAN_POINT('',(2.65,0.62,0.));
#15343=CARTESIAN_POINT('',(1.1,0.62,0.32));
#15344=CARTESIAN_POINT('',(1.1,0.62,0.16));
#15345=CARTESIAN_POINT('',(10.,0.62,0.32));
#15346=CARTESIAN_POINT('Origin',(-0.0999999999999996,0.62,0.32));
#15347=CARTESIAN_POINT('',(3.5,0.62,0.));
#15348=CARTESIAN_POINT('',(3.5,0.62,0.32));
#15349=CARTESIAN_POINT('',(3.5,0.62,0.16));
#15350=CARTESIAN_POINT('',(3.7,0.62,0.));
#15351=CARTESIAN_POINT('',(2.65,0.62,0.));
#15352=CARTESIAN_POINT('',(3.7,0.62,0.32));
#15353=CARTESIAN_POINT('',(3.7,0.62,0.16));
#15354=CARTESIAN_POINT('',(10.,0.62,0.32));
#15355=CARTESIAN_POINT('Origin',(4.95,0.,0.32));
#15356=CARTESIAN_POINT('',(1.6,-4.89858719658941E-17,0.32));
#15357=CARTESIAN_POINT('Origin',(2.,0.,0.32));
#15358=CARTESIAN_POINT('Origin',(4.95,0.,0.32));
#15359=CARTESIAN_POINT('',(8.4,-4.89858719658942E-17,0.32));
#15360=CARTESIAN_POINT('Origin',(8.8,0.,0.32));
#15361=CARTESIAN_POINT('Origin',(4.95,0.,0.32));
#15362=CARTESIAN_POINT('',(0.217044958570157,-0.7,0.32));
#15363=CARTESIAN_POINT('',(0.0167704893705731,-0.7,0.32));
#15364=CARTESIAN_POINT('Origin',(4.95,0.,0.32));
#15365=CARTESIAN_POINT('',(0.9,0.671641708581009,0.32));
#15366=CARTESIAN_POINT('',(1.1,-0.671641708581009,0.32));
#15367=CARTESIAN_POINT('Origin',(4.95,0.,0.32));
#15368=CARTESIAN_POINT('',(3.5,0.723888888888889,0.32));
#15369=CARTESIAN_POINT('',(3.7,-0.723888888888889,0.32));
#15370=CARTESIAN_POINT('Origin',(4.95,0.,0.32));
#15371=CARTESIAN_POINT('',(7.1,0.62,0.32));
#15372=CARTESIAN_POINT('',(7.1,0.712777777777778,0.32));
#15373=CARTESIAN_POINT('',(7.3,0.62,0.32));
#15374=CARTESIAN_POINT('',(10.,0.62,0.32));
#15375=CARTESIAN_POINT('',(7.3,-0.712777777777778,0.32));
#15376=CARTESIAN_POINT('Origin',(-0.0999999999999996,0.62,0.32));
#15377=CARTESIAN_POINT('',(7.1,0.62,0.));
#15378=CARTESIAN_POINT('',(7.1,0.62,0.16));
#15379=CARTESIAN_POINT('',(7.3,0.62,0.));
#15380=CARTESIAN_POINT('',(2.65,0.62,0.));
#15381=CARTESIAN_POINT('',(7.3,0.62,0.16));
#15382=CARTESIAN_POINT('Origin',(10.,1.30754691548544,0.));
#15383=CARTESIAN_POINT('',(10.,1.24211782565704,0.));
#15384=CARTESIAN_POINT('',(10.,-1.24211782565704,0.));
#15385=CARTESIAN_POINT('',(10.,1.30754691548544,0.));
#15386=CARTESIAN_POINT('',(10.,-1.20899340483173,0.605457329065657));
#15387=CARTESIAN_POINT('Ctrl Pts',(10.,-1.20899340483173,0.605457329065657));
#15388=CARTESIAN_POINT('Ctrl Pts',(10.,-1.21451837038612,0.504502771559899));
#15389=CARTESIAN_POINT('Ctrl Pts',(10.,-1.22004249263249,0.403547366186347));
#15390=CARTESIAN_POINT('Ctrl Pts',(10.,-1.23108392958594,0.201728789021226));
#15391=CARTESIAN_POINT('Ctrl Pts',(10.,-1.23660133320922,0.100864020914724));
#15392=CARTESIAN_POINT('Ctrl Pts',(10.,-1.24211782565704,0.));
#15393=CARTESIAN_POINT('Ctrl Pts',(10.,-1.10900986674273,0.7));
#15394=CARTESIAN_POINT('Ctrl Pts',(10.,-1.11692706738765,0.7));
#15395=CARTESIAN_POINT('Ctrl Pts',(9.99999896020971,-1.12478097169818,0.699006158364426));
#15396=CARTESIAN_POINT('Ctrl Pts',(9.99999805494427,-1.13243115645175,0.697118998397561));
#15397=CARTESIAN_POINT('Ctrl Pts',(9.99999754769332,-1.13671781459207,0.696061558623929));
#15398=CARTESIAN_POINT('Ctrl Pts',(9.99999708556116,-1.14094056283945,0.694722610426682));
#15399=CARTESIAN_POINT('Ctrl Pts',(9.99999679002998,-1.14507302265453,0.693112977943955));
#15400=CARTESIAN_POINT('Ctrl Pts',(9.99999625879002,-1.15250143622127,0.690219540062595));
#15401=CARTESIAN_POINT('Ctrl Pts',(9.999996365957,-1.15955821040664,0.686485807665162));
#15402=CARTESIAN_POINT('Ctrl Pts',(9.99999703387985,-1.16609707610076,0.681992895329386));
#15403=CARTESIAN_POINT('Ctrl Pts',(9.99999740034986,-1.16968476316425,0.679527763880215));
#15404=CARTESIAN_POINT('Ctrl Pts',(9.99999792190556,-1.17311627083768,0.676833210412541));
#15405=CARTESIAN_POINT('Ctrl Pts',(9.99999838578331,-1.17636354905877,0.673917165661822));
#15406=CARTESIAN_POINT('Ctrl Pts',(9.99999884023993,-1.17954487655573,0.671060344436104));
#15407=CARTESIAN_POINT('Ctrl Pts',(9.99999924462882,-1.18253006594632,0.668008218820746));
#15408=CARTESIAN_POINT('Ctrl Pts',(9.99999924442301,-1.185296421281,0.664772262763763));
#15409=CARTESIAN_POINT('Ctrl Pts',(9.99999924404215,-1.19041578560695,0.658783864313737));
#15410=CARTESIAN_POINT('Ctrl Pts',(9.99999800949836,-1.19478865237554,0.652167294255586));
#15411=CARTESIAN_POINT('Ctrl Pts',(9.99999759228052,-1.19835462180986,0.645087621913151));
#15412=CARTESIAN_POINT('Ctrl Pts',(9.99999755030119,-1.19871341999785,0.644375284453517));
#15413=CARTESIAN_POINT('Ctrl Pts',(9.9999975145836,-1.19906401030029,0.643658239626438));
#15414=CARTESIAN_POINT('Ctrl Pts',(9.99999748581823,-1.19940630408966,0.642936645100882));
#15415=CARTESIAN_POINT('Ctrl Pts',(9.99999720003888,-1.20280693749908,0.635767720253638));
#15416=CARTESIAN_POINT('Ctrl Pts',(9.9999978299417,-1.20535324884233,0.628234501710241));
#15417=CARTESIAN_POINT('Ctrl Pts',(9.99999874867777,-1.20699142055415,0.62050509267719));
#15418=CARTESIAN_POINT('Ctrl Pts',(9.99999933690345,-1.20804026874419,0.615556297251186));
#15419=CARTESIAN_POINT('Ctrl Pts',(9.99999999916487,-1.20871598809812,0.61052641213707));
#15420=CARTESIAN_POINT('Ctrl Pts',(9.99999999968202,-1.20899340489109,0.605457329065633));
#15421=CARTESIAN_POINT('Ctrl Pts',(10.,1.24211782565704,0.));
#15422=CARTESIAN_POINT('Ctrl Pts',(10.,1.23660053043673,0.100878698875723));
#15423=CARTESIAN_POINT('Ctrl Pts',(10.,1.23108232376984,0.201758145268796));
#15424=CARTESIAN_POINT('Ctrl Pts',(10.,1.22004088630648,0.403576722396156));
#15425=CARTESIAN_POINT('Ctrl Pts',(10.,1.2145175671044,0.504517449470448));
#15426=CARTESIAN_POINT('Ctrl Pts',(10.,1.20899340483173,0.605457329065657));
#15427=CARTESIAN_POINT('Origin',(7.3,-1.42555555555556,0.));
#15428=CARTESIAN_POINT('',(7.3,1.35236351479115,0.));
#15429=CARTESIAN_POINT('',(7.3,-1.42555555555556,0.));
#15430=CARTESIAN_POINT('Ctrl Pts',(7.29999999953133,1.3203161347307,0.605285370449834));
#15431=CARTESIAN_POINT('Ctrl Pts',(7.29999999953133,1.32565322760551,0.504490726585133));
#15432=CARTESIAN_POINT('Ctrl Pts',(7.3,1.33099015509697,0.403695123734478));
#15433=CARTESIAN_POINT('Ctrl Pts',(7.3,1.34167258064689,0.201933969199042));
#15434=CARTESIAN_POINT('Ctrl Pts',(7.3,1.34701817868136,0.100966514951419));
#15435=CARTESIAN_POINT('Ctrl Pts',(7.3,1.35236351479115,0.));
#15436=CARTESIAN_POINT('',(7.29999999953133,-1.3203161347307,0.605285370449834));
#15437=CARTESIAN_POINT('Ctrl Pts',(7.3,-1.32031613470337,0.605285370449877));
#15438=CARTESIAN_POINT('Ctrl Pts',(7.3,-1.31989712778929,0.61319860217968));
#15439=CARTESIAN_POINT('Ctrl Pts',(7.29999916171872,-1.31851071739963,0.621020829077898));
#15440=CARTESIAN_POINT('Ctrl Pts',(7.29999878808195,-1.31624092632926,0.628591660945423));
#15441=CARTESIAN_POINT('Ctrl Pts',(7.29999857947278,-1.31497365483497,0.632818613610392));
#15442=CARTESIAN_POINT('Ctrl Pts',(7.29999848639856,-1.31343001415,0.636967235874856));
#15443=CARTESIAN_POINT('Ctrl Pts',(7.29999853830689,-1.31161789606625,0.641007613679984));
#15444=CARTESIAN_POINT('Ctrl Pts',(7.29999863125487,-1.30837308502546,0.648242386418365));
#15445=CARTESIAN_POINT('Ctrl Pts',(7.29999925734287,-1.30430566789097,0.655052076019481));
#15446=CARTESIAN_POINT('Ctrl Pts',(7.29999949821933,-1.29947941328181,0.661273460789274));
#15447=CARTESIAN_POINT('Ctrl Pts',(7.29999954322,-1.29857776968225,0.662435743389828));
#15448=CARTESIAN_POINT('Ctrl Pts',(7.29999957102613,-1.29764951297213,0.663577423078133));
#15449=CARTESIAN_POINT('Ctrl Pts',(7.2999995707084,-1.29669488998092,0.664697318929248));
#15450=CARTESIAN_POINT('Ctrl Pts',(7.29999957007561,-1.29479368240016,0.666927680549918));
#15451=CARTESIAN_POINT('Ctrl Pts',(7.29999945886743,-1.29278792931167,0.669071688571899));
#15452=CARTESIAN_POINT('Ctrl Pts',(7.29999930790078,-1.2906849717248,0.671125563583336));
#15453=CARTESIAN_POINT('Ctrl Pts',(7.29999889984047,-1.28500071247856,0.676677153447665));
#15454=CARTESIAN_POINT('Ctrl Pts',(7.29999826931494,-1.27867319504519,0.681510485910933));
#15455=CARTESIAN_POINT('Ctrl Pts',(7.29999806345125,-1.27186607945067,0.685571085769401));
#15456=CARTESIAN_POINT('Ctrl Pts',(7.29999793266427,-1.26754145993833,0.688150820039508));
#15457=CARTESIAN_POINT('Ctrl Pts',(7.29999794545359,-1.26302231037287,0.690417984675215));
#15458=CARTESIAN_POINT('Ctrl Pts',(7.29999810371711,-1.25834494218995,0.69234933099425));
#15459=CARTESIAN_POINT('Ctrl Pts',(7.29999835129001,-1.25102809722258,0.695370551698293));
#15460=CARTESIAN_POINT('Ctrl Pts',(7.29999895574222,-1.24340909242398,0.6975375590939));
#15461=CARTESIAN_POINT('Ctrl Pts',(7.29999944081525,-1.2356348173965,0.698780605629559));
#15462=CARTESIAN_POINT('Ctrl Pts',(7.29999975409932,-1.23061380764338,0.699583426311495));
#15463=CARTESIAN_POINT('Ctrl Pts',(7.30000000047446,-1.22552743956586,0.699999999832051));
#15464=CARTESIAN_POINT('Ctrl Pts',(7.29999999989087,-1.22041345054982,0.7));
#15465=CARTESIAN_POINT('',(7.3,-1.35236351479115,0.));
#15466=CARTESIAN_POINT('Ctrl Pts',(7.3,-1.35236351479115,0.));
#15467=CARTESIAN_POINT('Ctrl Pts',(7.3,-1.34701814920095,0.100967071798286));
#15468=CARTESIAN_POINT('Ctrl Pts',(7.3,-1.34167252169398,0.201935082699409));
#15469=CARTESIAN_POINT('Ctrl Pts',(7.3,-1.33099009614589,0.403696237111114));
#15470=CARTESIAN_POINT('Ctrl Pts',(7.29999999953133,-1.32565319812959,0.504491283257837));
#15471=CARTESIAN_POINT('Ctrl Pts',(7.29999999953133,-1.3203161347307,0.605285370449834));
#15472=CARTESIAN_POINT('',(7.3,-1.42555555555556,0.));
#15473=CARTESIAN_POINT('Origin',(3.7,-1.44777777777778,0.));
#15474=CARTESIAN_POINT('',(3.7,1.37924639543935,0.));
#15475=CARTESIAN_POINT('',(3.7,-1.44777777777778,0.));
#15476=CARTESIAN_POINT('',(3.7,1.34735368793805,0.605261457205193));
#15477=CARTESIAN_POINT('Ctrl Pts',(3.7,1.34735368793805,0.605261457205193));
#15478=CARTESIAN_POINT('Ctrl Pts',(3.7,1.35266395147774,0.504488703431434));
#15479=CARTESIAN_POINT('Ctrl Pts',(3.7,1.35797406404029,0.40371594170176));
#15480=CARTESIAN_POINT('Ctrl Pts',(3.7,1.36860496587027,0.201962122597264));
#15481=CARTESIAN_POINT('Ctrl Pts',(3.7,1.37392575452088,0.100981065191366));
#15482=CARTESIAN_POINT('Ctrl Pts',(3.7,1.37924639543935,0.));
#15483=CARTESIAN_POINT('',(3.7,1.24747724070879,0.7));
#15484=CARTESIAN_POINT('Ctrl Pts',(3.7,1.24747724070879,0.7));
#15485=CARTESIAN_POINT('Ctrl Pts',(3.7,1.25538532734776,0.7));
#15486=CARTESIAN_POINT('Ctrl Pts',(3.70000034866643,1.26322972530331,0.699006048248363));
#15487=CARTESIAN_POINT('Ctrl Pts',(3.70000065268588,1.27087026624727,0.697119044026295));
#15488=CARTESIAN_POINT('Ctrl Pts',(3.7000008238479,1.27517186762995,0.696056666371322));
#15489=CARTESIAN_POINT('Ctrl Pts',(3.70000097972585,1.27940891103121,0.694710185093394));
#15490=CARTESIAN_POINT('Ctrl Pts',(3.70000107833511,1.28355469746902,0.693090631030141));
#15491=CARTESIAN_POINT('Ctrl Pts',(3.70000125487464,1.29097687270382,0.690191153635441));
#15492=CARTESIAN_POINT('Ctrl Pts',(3.7000012145424,1.29802606517866,0.686451118058958));
#15493=CARTESIAN_POINT('Ctrl Pts',(3.70000098691147,1.3045562506385,0.681952404110064));
#15494=CARTESIAN_POINT('Ctrl Pts',(3.70000086156653,1.30815209635338,0.679475187900035));
#15495=CARTESIAN_POINT('Ctrl Pts',(3.70000068390876,1.31159030769532,0.676767042898431));
#15496=CARTESIAN_POINT('Ctrl Pts',(3.70000052608992,1.31484259178137,0.673836088143417));
#15497=CARTESIAN_POINT('Ctrl Pts',(3.70000037216713,1.31801458722906,0.670977489418868));
#15498=CARTESIAN_POINT('Ctrl Pts',(3.70000023558528,1.32099045552882,0.667924239810466));
#15499=CARTESIAN_POINT('Ctrl Pts',(3.70000023595245,1.32374763345498,0.664687876924229));
#15500=CARTESIAN_POINT('Ctrl Pts',(3.70000023663259,1.32885491153898,0.658692977181302));
#15501=CARTESIAN_POINT('Ctrl Pts',(3.70000065621025,1.33321474659758,0.652071180203097));
#15502=CARTESIAN_POINT('Ctrl Pts',(3.70000080093706,1.33676785491319,0.644988218508662));
#15503=CARTESIAN_POINT('Ctrl Pts',(3.70000081573428,1.33713113341147,0.644264039153811));
#15504=CARTESIAN_POINT('Ctrl Pts',(3.70000082835625,1.33748593861467,0.643535019157411));
#15505=CARTESIAN_POINT('Ctrl Pts',(3.70000083855542,1.33783217873901,0.642801324492746));
#15506=CARTESIAN_POINT('Ctrl Pts',(3.70000093832019,1.34121897990539,0.63562457699476));
#15507=CARTESIAN_POINT('Ctrl Pts',(3.70000072997693,1.34375116782692,0.628085030530103));
#15508=CARTESIAN_POINT('Ctrl Pts',(3.70000042189378,1.34537558692779,0.6203512574804));
#15509=CARTESIAN_POINT('Ctrl Pts',(3.70000022417294,1.3464181026242,0.615387895628485));
#15510=CARTESIAN_POINT('Ctrl Pts',(3.70000000036652,1.34708586836718,0.6103438638189));
#15511=CARTESIAN_POINT('Ctrl Pts',(3.69999999992214,1.34735368792773,0.6052614572053));
#15512=CARTESIAN_POINT('',(3.7,-1.24747724070944,0.7));
#15513=CARTESIAN_POINT('',(3.7,-0.723888888888889,0.7));
#15514=CARTESIAN_POINT('',(3.7,-1.34735368793805,0.605261457205193));
#15515=CARTESIAN_POINT('Ctrl Pts',(3.69999999992215,-1.34735368792773,0.6052614572053));
#15516=CARTESIAN_POINT('Ctrl Pts',(3.70000000061408,-1.34693666923469,0.613175212866596));
#15517=CARTESIAN_POINT('Ctrl Pts',(3.70000049671034,-1.34555248374866,0.620998392122869));
#15518=CARTESIAN_POINT('Ctrl Pts',(3.70000071566022,-1.34328499565267,0.628570462735333));
#15519=CARTESIAN_POINT('Ctrl Pts',(3.70000083807517,-1.34201724238155,0.632804009674372));
#15520=CARTESIAN_POINT('Ctrl Pts',(3.7000008913247,-1.34047237297042,0.63695909738719));
#15521=CARTESIAN_POINT('Ctrl Pts',(3.70000085837557,-1.33865827982058,0.641005656934072));
#15522=CARTESIAN_POINT('Ctrl Pts',(3.7000007994669,-1.33541492172585,0.648240369034365));
#15523=CARTESIAN_POINT('Ctrl Pts',(3.70000042420685,-1.33134915897915,0.655050234746405));
#15524=CARTESIAN_POINT('Ctrl Pts',(3.70000027984635,-1.32652447879733,0.661271863919233));
#15525=CARTESIAN_POINT('Ctrl Pts',(3.70000025294096,-1.32562527203035,0.662431429080655));
#15526=CARTESIAN_POINT('Ctrl Pts',(3.7000002362737,-1.32469957579387,0.663570491348455));
#15527=CARTESIAN_POINT('Ctrl Pts',(3.70000023630138,-1.32374763346102,0.664687876924223));
#15528=CARTESIAN_POINT('Ctrl Pts',(3.70000023635686,-1.32184039796576,0.666926581264246));
#15529=CARTESIAN_POINT('Ctrl Pts',(3.70000030283857,-1.31982784222224,0.669078323867587));
#15530=CARTESIAN_POINT('Ctrl Pts',(3.70000039320883,-1.31771738411303,0.671139279696989));
#15531=CARTESIAN_POINT('Ctrl Pts',(3.70000063660146,-1.3120333248939,0.676690015307994));
#15532=CARTESIAN_POINT('Ctrl Pts',(3.7000010126336,-1.30570602994251,0.681522474044465));
#15533=CARTESIAN_POINT('Ctrl Pts',(3.70000113724274,-1.29889910811053,0.685582059356066));
#15534=CARTESIAN_POINT('Ctrl Pts',(3.70000121634872,-1.29457784995583,0.688159217808216));
#15535=CARTESIAN_POINT('Ctrl Pts',(3.70000121058612,-1.2900623422215,0.690424215862126));
#15536=CARTESIAN_POINT('Ctrl Pts',(3.70000111831253,-1.28538881676413,0.692353818784707));
#15537=CARTESIAN_POINT('Ctrl Pts',(3.70000097388434,-1.27807373536961,0.695374066040565));
#15538=CARTESIAN_POINT('Ctrl Pts',(3.70000061691996,-1.27045659963863,0.697540160564298));
#15539=CARTESIAN_POINT('Ctrl Pts',(3.7000003304055,-1.26268427129293,0.698782316368755));
#15540=CARTESIAN_POINT('Ctrl Pts',(3.70000014548661,-1.25766794365683,0.699584014420239));
#15541=CARTESIAN_POINT('Ctrl Pts',(3.7,-1.25258637988459,0.7));
#15542=CARTESIAN_POINT('Ctrl Pts',(3.7,-1.24747724070879,0.7));
#15543=CARTESIAN_POINT('',(3.7,-1.37924639543935,0.));
#15544=CARTESIAN_POINT('Ctrl Pts',(3.7,-1.37924639543935,0.));
#15545=CARTESIAN_POINT('Ctrl Pts',(3.7,-1.37392574223662,0.100981298335747));
#15546=CARTESIAN_POINT('Ctrl Pts',(3.7,-1.36860494130098,0.201962588887634));
#15547=CARTESIAN_POINT('Ctrl Pts',(3.7,-1.35797403946962,0.403716407992068));
#15548=CARTESIAN_POINT('Ctrl Pts',(3.7,-1.3526639391921,0.504488936575732));
#15549=CARTESIAN_POINT('Ctrl Pts',(3.7,-1.34735368793805,0.605261457205193));
#15550=CARTESIAN_POINT('',(3.7,-1.44777777777778,0.));
#15551=CARTESIAN_POINT('Origin',(1.1,-1.34328341716202,0.));
#15552=CARTESIAN_POINT('',(1.1,1.27885335043294,0.));
#15553=CARTESIAN_POINT('',(1.1,-1.34328341716202,0.));
#15554=CARTESIAN_POINT('Ctrl Pts',(1.1,1.24553911298206,0.605485603995113));
#15555=CARTESIAN_POINT('Ctrl Pts',(1.1,1.25109559382646,0.504544105903265));
#15556=CARTESIAN_POINT('Ctrl Pts',(1.1,1.25665083308595,0.403601248768354));
#15557=CARTESIAN_POINT('Ctrl Pts',(1.1,1.26775551906787,0.201773573764085));
#15558=CARTESIAN_POINT('Ctrl Pts',(1.1,1.2733051088238,0.100886182270816));
#15559=CARTESIAN_POINT('Ctrl Pts',(1.1,1.27885335043294,0.));
#15560=CARTESIAN_POINT('',(1.1,-1.14549341399195,0.7));
#15561=CARTESIAN_POINT('',(1.1,-0.671641708581009,0.7));
#15562=CARTESIAN_POINT('',(1.1,-1.24553911298206,0.605485603995113));
#15563=CARTESIAN_POINT('Ctrl Pts',(1.09999999916631,-1.24553911263843,0.605485603997431));
#15564=CARTESIAN_POINT('Ctrl Pts',(1.10000000220634,-1.24510362317222,0.61339691285734));
#15565=CARTESIAN_POINT('Ctrl Pts',(1.10000177015643,-1.24370036622144,0.621215229994996));
#15566=CARTESIAN_POINT('Ctrl Pts',(1.10000252895322,-1.24141353486351,0.628780213666851));
#15567=CARTESIAN_POINT('Ctrl Pts',(1.10000294802756,-1.24015054543059,0.632958263090869));
#15568=CARTESIAN_POINT('Ctrl Pts',(1.10000312162076,-1.23861706177488,0.637059070655947));
#15569=CARTESIAN_POINT('Ctrl Pts',(1.10000299297862,-1.23682078380192,0.641053713130525));
#15570=CARTESIAN_POINT('Ctrl Pts',(1.10000275999609,-1.23356756237267,0.64828837095969));
#15571=CARTESIAN_POINT('Ctrl Pts',(1.10000138715103,-1.22949085733774,0.655096441442141));
#15572=CARTESIAN_POINT('Ctrl Pts',(1.10000084482056,-1.2246552743941,0.661315040399663));
#15573=CARTESIAN_POINT('Ctrl Pts',(1.10000074196669,-1.22373819809959,0.662494407966206));
#15574=CARTESIAN_POINT('Ctrl Pts',(1.1000006773267,-1.22279369438101,0.663652502541609));
#15575=CARTESIAN_POINT('Ctrl Pts',(1.10000067553493,-1.22182202641035,0.66478809188211));
#15576=CARTESIAN_POINT('Ctrl Pts',(1.10000067210542,-1.219962222636,0.666961646435043));
#15577=CARTESIAN_POINT('Ctrl Pts',(1.10000089707048,-1.21800293160495,0.669052796220007));
#15578=CARTESIAN_POINT('Ctrl Pts',(1.10000120920309,-1.21595100691259,0.671058078730413));
#15579=CARTESIAN_POINT('Ctrl Pts',(1.10000207391986,-1.21026645613745,0.676613414309409));
#15580=CARTESIAN_POINT('Ctrl Pts',(1.1000034579227,-1.20393786500476,0.681450029097565));
#15581=CARTESIAN_POINT('Ctrl Pts',(1.10000394126019,-1.19712964857754,0.685514663758263));
#15582=CARTESIAN_POINT('Ctrl Pts',(1.10000424974863,-1.19278432848208,0.688108902478585));
#15583=CARTESIAN_POINT('Ctrl Pts',(1.10000425197701,-1.18824265871575,0.690387991283085));
#15584=CARTESIAN_POINT('Ctrl Pts',(1.10000394032285,-1.18354156621637,0.692328715646671));
#15585=CARTESIAN_POINT('Ctrl Pts',(1.10000345443802,-1.17621232165581,0.695354404566264));
#15586=CARTESIAN_POINT('Ctrl Pts',(1.10000219938511,-1.16858027633095,0.697525330589554));
#15587=CARTESIAN_POINT('Ctrl Pts',(1.10000118192936,-1.16079305972554,0.698772417158578));
#15588=CARTESIAN_POINT('Ctrl Pts',(1.10000052251962,-1.15574619011492,0.699580649884844));
#15589=CARTESIAN_POINT('Ctrl Pts',(1.1,-1.15063354328712,0.7));
#15590=CARTESIAN_POINT('Ctrl Pts',(1.1,-1.14549341399196,0.7));
#15591=CARTESIAN_POINT('',(1.1,-1.27885335043294,0.));
#15592=CARTESIAN_POINT('Ctrl Pts',(1.1,-1.27885335043294,0.));
#15593=CARTESIAN_POINT('Ctrl Pts',(1.1,-1.27330503870861,0.100887457206881));
#15594=CARTESIAN_POINT('Ctrl Pts',(1.1,-1.26775537880223,0.201776123688554));
#15595=CARTESIAN_POINT('Ctrl Pts',(1.1,-1.25665069275548,0.403603798678134));
#15596=CARTESIAN_POINT('Ctrl Pts',(1.1,-1.25109552364596,0.504545380833391));
#15597=CARTESIAN_POINT('Ctrl Pts',(1.1,-1.24553911298206,0.605485603995113));
#15598=CARTESIAN_POINT('',(1.1,-1.34328341716202,0.));
#15599=CARTESIAN_POINT('Origin',(0.199725906950915,-1.4,-0.0104671912485888));
#15600=CARTESIAN_POINT('',(0.200274469199584,1.12301388185427,1.38777878078145E-17));
#15601=CARTESIAN_POINT('',(0.200274469199585,-0.7,0.));
#15602=CARTESIAN_POINT('',(0.231993417893744,1.09142177001972,0.605233595624295));
#15603=CARTESIAN_POINT('Ctrl Pts',(0.200274469199584,1.12301388185427,-2.97071395261028E-17));
#15604=CARTESIAN_POINT('Ctrl Pts',(0.210847451470635,1.11248294808,0.201744519910852));
#15605=CARTESIAN_POINT('Ctrl Pts',(0.22142043436526,1.101952242875,0.403489051720196));
#15606=CARTESIAN_POINT('Ctrl Pts',(0.231993417893744,1.09142177001972,0.605233595624295));
#15607=CARTESIAN_POINT('',(0.231993417893744,-1.09142177001972,0.605233595624295));
#15608=CARTESIAN_POINT('',(0.231993417893744,-0.7,0.605233595624295));
#15609=CARTESIAN_POINT('',(0.200274469199584,-1.12301388185427,-1.38777878078145E-17));
#15610=CARTESIAN_POINT('Ctrl Pts',(0.231993417893744,-1.09142177001972,
0.605233595624295));
#15611=CARTESIAN_POINT('Ctrl Pts',(0.22142043436526,-1.101952242875,0.403489051720196));
#15612=CARTESIAN_POINT('Ctrl Pts',(0.210847451470635,-1.11248294808,0.201744519910852));
#15613=CARTESIAN_POINT('Ctrl Pts',(0.200274469199584,-1.12301388185427,
-4.90059381963448E-17));
#15614=CARTESIAN_POINT('',(0.200274469199585,-0.7,0.));
#15615=CARTESIAN_POINT('Origin',(5.4,-1.11022302462516E-16,0.));
#15616=CARTESIAN_POINT('Ctrl Pts',(7.29999999999999,-1.35236351479115,1.04083408558608E-17));
#15617=CARTESIAN_POINT('Ctrl Pts',(8.20044803681595,-1.32637404707459,3.18306896032855E-8));
#15618=CARTESIAN_POINT('Ctrl Pts',(9.10060048441536,-1.28803709316692,1.03188250195688E-8));
#15619=CARTESIAN_POINT('Ctrl Pts',(10.0000000000405,-1.24211782537639,-8.23328475353175E-12));
#15620=CARTESIAN_POINT('Ctrl Pts',(10.0000000000405,1.24211782537639,-8.23320567538283E-12));
#15621=CARTESIAN_POINT('Ctrl Pts',(9.1006004808701,1.28803709334794,1.03184817085883E-8));
#15622=CARTESIAN_POINT('Ctrl Pts',(8.20044803144508,1.32637404722969,3.18291413954212E-8));
#15623=CARTESIAN_POINT('Ctrl Pts',(7.3,1.35236351479115,4.75121773919879E-17));
#15624=CARTESIAN_POINT('',(7.1,1.35793097395724,0.));
#15625=CARTESIAN_POINT('',(7.1,1.42555555555556,0.));
#15626=CARTESIAN_POINT('Ctrl Pts',(7.1000000000396,1.35793097389613,-4.88924676637329E-12));
#15627=CARTESIAN_POINT('Ctrl Pts',(6.53177385320612,1.37316067096195,3.71763852401782E-9));
#15628=CARTESIAN_POINT('Ctrl Pts',(5.96344379069665,1.38333257666104,-3.82408184804385E-8));
#15629=CARTESIAN_POINT('Ctrl Pts',(5.39512359652123,1.38725406840392,-3.97623797275691E-8));
#15630=CARTESIAN_POINT('Ctrl Pts',(4.82973248928002,1.39115534902226,-4.12760989429076E-8));
#15631=CARTESIAN_POINT('Ctrl Pts',(4.26470859812609,1.38886839226708,1.63957607983357E-8));
#15632=CARTESIAN_POINT('Ctrl Pts',(3.70000000036239,1.37924639538501,-6.25376529969227E-12));
#15633=CARTESIAN_POINT('',(3.5,1.37552980833516,0.));
#15634=CARTESIAN_POINT('',(3.5,1.44777777777778,0.));
#15635=CARTESIAN_POINT('Ctrl Pts',(3.50000000097466,1.37552980835479,1.06251812903579E-15));
#15636=CARTESIAN_POINT('Ctrl Pts',(2.69943075695685,1.35940904975719,2.35366119539541E-7));
#15637=CARTESIAN_POINT('Ctrl Pts',(1.89948254587541,1.32827224396921,2.51300192353997E-7));
#15638=CARTESIAN_POINT('Ctrl Pts',(1.10000000028363,1.27885335028943,-5.13283415455519E-11));
#15639=CARTESIAN_POINT('',(0.9,1.266106713614,0.));
#15640=CARTESIAN_POINT('',(0.9,1.34328341716202,0.));
#15641=CARTESIAN_POINT('',(0.292382661757373,1.22257596919059,0.));
#15642=CARTESIAN_POINT('Ctrl Pts',(0.9,1.266106713614,1.20346441145891E-16));
#15643=CARTESIAN_POINT('Ctrl Pts',(0.697432754539207,1.25280566772398,-2.10387859372414E-8));
#15644=CARTESIAN_POINT('Ctrl Pts',(0.494894520889663,1.23831317328004,3.6654767345328E-12));
#15645=CARTESIAN_POINT('Ctrl Pts',(0.292382661757371,1.22257596919059,2.98331735103528E-16));
#15646=CARTESIAN_POINT('Ctrl Pts',(0.292382661757373,1.22257596919059,2.94902990916057E-17));
#15647=CARTESIAN_POINT('Ctrl Pts',(0.284469747869226,1.22196105627757,-8.65621238729993E-13));
#15648=CARTESIAN_POINT('Ctrl Pts',(0.276673396002317,1.22038240716686,-1.19564355630166E-6));
#15649=CARTESIAN_POINT('Ctrl Pts',(0.269153172408756,1.21792571627104,-1.29137975931779E-6));
#15650=CARTESIAN_POINT('Ctrl Pts',(0.264330998492885,1.21635041859408,-1.35276844214688E-6));
#15651=CARTESIAN_POINT('Ctrl Pts',(0.259622238853914,1.21441292414196,-1.0165784587106E-6));
#15652=CARTESIAN_POINT('Ctrl Pts',(0.255072584042237,1.21212521597766,-4.21167369976509E-7));
#15653=CARTESIAN_POINT('Ctrl Pts',(0.247984787860257,1.20856125126747,5.06409032217246E-7));
#15654=CARTESIAN_POINT('Ctrl Pts',(0.241364979299678,1.20419126978451,2.25366520907849E-6));
#15655=CARTESIAN_POINT('Ctrl Pts',(0.235375785094684,1.19908071490398,1.28723124315333E-6));
#15656=CARTESIAN_POINT('Ctrl Pts',(0.235058634311792,1.19881009144014,1.23605486142058E-6));
#15657=CARTESIAN_POINT('Ctrl Pts',(0.234743258170683,1.19853738091759,1.17639378419006E-6));
#15658=CARTESIAN_POINT('Ctrl Pts',(0.234429683218046,1.19826258967301,1.10742116603597E-6));
#15659=CARTESIAN_POINT('Ctrl Pts',(0.23095881299434,1.19522100506769,3.4398325561458E-7));
#15660=CARTESIAN_POINT('Ctrl Pts',(0.227708211416394,1.19192479473749,-1.52348441667556E-6));
#15661=CARTESIAN_POINT('Ctrl Pts',(0.224692430858345,1.18840300965977,-3.42436181452249E-6));
#15662=CARTESIAN_POINT('Ctrl Pts',(0.219522873151367,1.18236607466387,-6.68278702580898E-6));
#15663=CARTESIAN_POINT('Ctrl Pts',(0.21509942609515,1.17573654654733,-9.78259773483875E-6));
#15664=CARTESIAN_POINT('Ctrl Pts',(0.211478909386775,1.16867548752938,-1.04320859863301E-5));
#15665=CARTESIAN_POINT('Ctrl Pts',(0.20968494559888,1.16517673715679,-1.075390701291E-5));
#15666=CARTESIAN_POINT('Ctrl Pts',(0.208088728862602,1.16157146972622,-1.05358292927083E-5));
#15667=CARTESIAN_POINT('Ctrl Pts',(0.206701335101202,1.15787708229469,-9.83193564179307E-6));
#15668=CARTESIAN_POINT('Ctrl Pts',(0.203919119965097,1.15046852899383,-8.42037994342582E-6));
#15669=CARTESIAN_POINT('Ctrl Pts',(0.202003457218558,1.1427818296106,-4.88542801801716E-6));
#15670=CARTESIAN_POINT('Ctrl Pts',(0.201024541128784,1.13496408391561,-2.30807221316776E-6));
#15671=CARTESIAN_POINT('Ctrl Pts',(0.200529226009753,1.13100843574523,-1.00397341389412E-6));
#15672=CARTESIAN_POINT('Ctrl Pts',(0.200274469344113,1.12701892049093,-1.14168925800036E-11));
#15673=CARTESIAN_POINT('Ctrl Pts',(0.200274469199584,1.12301388185427,-1.43114686768087E-17));
#15674=CARTESIAN_POINT('',(-1.73234772679968E-18,1.12356026268968,4.53319947845445E-20));
#15675=CARTESIAN_POINT('',(0.,-1.4,0.));
#15676=CARTESIAN_POINT('',(0.276326924564679,1.42224670711126,-2.77555756156289E-17));
#15677=CARTESIAN_POINT('Ctrl Pts',(0.276326924564681,1.42224670711126,-1.50920942409982E-16));
#15678=CARTESIAN_POINT('Ctrl Pts',(0.258529852003869,1.4208638358667,-3.32972379743633E-13));
#15679=CARTESIAN_POINT('Ctrl Pts',(0.240927013527826,1.41785398988725,-1.99727536601662E-6));
#15680=CARTESIAN_POINT('Ctrl Pts',(0.223720619657732,1.41333325652174,-2.71091968639774E-6));
#15681=CARTESIAN_POINT('Ctrl Pts',(0.206313289378911,1.40875972999491,-3.432897951005E-6));
#15682=CARTESIAN_POINT('Ctrl Pts',(0.18931019325249,1.40263932318529,-2.78724979559428E-6));
#15683=CARTESIAN_POINT('Ctrl Pts',(0.172932985028856,1.39504220432096,-6.31841720307455E-7));
#15684=CARTESIAN_POINT('Ctrl Pts',(0.170060146426803,1.39370954151055,-2.53746782677961E-7));
#15685=CARTESIAN_POINT('Ctrl Pts',(0.167206630967902,1.39233132643846,1.61597591574489E-7));
#15686=CARTESIAN_POINT('Ctrl Pts',(0.164373729059928,1.39090779908693,6.02790108062464E-7));
#15687=CARTESIAN_POINT('Ctrl Pts',(0.148213121449433,1.38278712717586,3.11962244863226E-6));
#15688=CARTESIAN_POINT('Ctrl Pts',(0.132864864406694,1.37326763401578,6.8005293729143E-6));
#15689=CARTESIAN_POINT('Ctrl Pts',(0.118540368157823,1.36244192017091,7.47011412280372E-6));
#15690=CARTESIAN_POINT('Ctrl Pts',(0.1130124780146,1.35826422653222,7.72851001154276E-6));
#15691=CARTESIAN_POINT('Ctrl Pts',(0.107637267132642,1.35389150739715,7.50091387420595E-6));
#15692=CARTESIAN_POINT('Ctrl Pts',(0.102427993107927,1.34932731552598,6.39696583889361E-6));
#15693=CARTESIAN_POINT('Ctrl Pts',(0.0920147884934566,1.34020361352282,
4.19020214765608E-6));
#15694=CARTESIAN_POINT('Ctrl Pts',(0.082263696775192,1.33031540618347,-1.43705507633734E-6));
#15695=CARTESIAN_POINT('Ctrl Pts',(0.0732179607829324,1.31975004019149,
-7.24116446069057E-6));
#15696=CARTESIAN_POINT('Ctrl Pts',(0.0614369648181435,1.30598990677343,
-1.48003270644599E-5));
#15697=CARTESIAN_POINT('Ctrl Pts',(0.0509520748529884,1.29120077200215,
-2.24515165560165E-5));
#15698=CARTESIAN_POINT('Ctrl Pts',(0.0418305631051555,1.27560026299671,
-2.64881615939377E-5));
#15699=CARTESIAN_POINT('Ctrl Pts',(0.0329966685655992,1.26049166530727,
-3.03975241584371E-5));
#15700=CARTESIAN_POINT('Ctrl Pts',(0.0254411283904758,1.24462062939249,
-3.09701348507133E-5));
#15701=CARTESIAN_POINT('Ctrl Pts',(0.0192647836588538,1.2281607987719,-2.81763116144976E-5));
#15702=CARTESIAN_POINT('Ctrl Pts',(0.0129258683931997,1.2112677210496,-2.53089508159798E-5));
#15703=CARTESIAN_POINT('Ctrl Pts',(0.00809110271874438,1.19389182855556,
-1.89493195503086E-5));
#15704=CARTESIAN_POINT('Ctrl Pts',(0.00484442764459327,1.17622983835018,
-1.25518552566888E-5));
#15705=CARTESIAN_POINT('Ctrl Pts',(0.00165723550742335,1.1588914367474,
-6.27160009448058E-6));
#15706=CARTESIAN_POINT('Ctrl Pts',(1.90718451428807E-9,1.14127598190669,
-1.51296892603399E-10));
#15707=CARTESIAN_POINT('Ctrl Pts',(2.41777084464267E-17,1.12356026268968,
-3.46944695195361E-18));
#15708=CARTESIAN_POINT('',(10.5166159648474,1.4155315881283,0.));
#15709=CARTESIAN_POINT('Ctrl Pts',(0.276326924564679,1.42224670711126,0.));
#15710=CARTESIAN_POINT('Ctrl Pts',(3.68975660465893,1.68747752195839,0.));
#15711=CARTESIAN_POINT('Ctrl Pts',(7.10318628475318,1.599994843061,0.));
#15712=CARTESIAN_POINT('Ctrl Pts',(10.5166159648474,1.4155315881283,0.));
#15713=CARTESIAN_POINT('',(10.8,1.11638029377732,-5.56631991785941E-17));
#15714=CARTESIAN_POINT('Ctrl Pts',(10.8,1.11638029377732,2.32452945780892E-16));
#15715=CARTESIAN_POINT('Ctrl Pts',(10.7999999994302,1.13421844616111,-9.29296349749781E-12));
#15716=CARTESIAN_POINT('Ctrl Pts',(10.7983603663884,1.15198349698667,-2.38856955364628E-6));
#15717=CARTESIAN_POINT('Ctrl Pts',(10.7951843826221,1.16946861094468,-3.77014304120448E-6));
#15718=CARTESIAN_POINT('Ctrl Pts',(10.7919669771209,1.18718176881198,-5.16973525142236E-6));
#15719=CARTESIAN_POINT('Ctrl Pts',(10.7871724978816,1.20460918321158,-5.4755482503851E-6));
#15720=CARTESIAN_POINT('Ctrl Pts',(10.7808573412527,1.22152732075962,-4.27334038376583E-6));
#15721=CARTESIAN_POINT('Ctrl Pts',(10.7797421066656,1.22451500471617,-4.06103467663179E-6));
#15722=CARTESIAN_POINT('Ctrl Pts',(10.7785793293545,1.22748675045939,-3.81081650224554E-6));
#15723=CARTESIAN_POINT('Ctrl Pts',(10.7773691713543,1.23044124224994,-3.53261416912234E-6));
#15724=CARTESIAN_POINT('Ctrl Pts',(10.7705159051166,1.24717287467681,-1.95712183132163E-6));
#15725=CARTESIAN_POINT('Ctrl Pts',(10.7622076549587,1.26320448426569,8.50150473021234E-7));
#15726=CARTESIAN_POINT('Ctrl Pts',(10.7525236566209,1.27832128496499,1.09915986206012E-6));
#15727=CARTESIAN_POINT('Ctrl Pts',(10.7482509716548,1.28499098118248,1.20902550183604E-6));
#15728=CARTESIAN_POINT('Ctrl Pts',(10.7437098328292,1.29148238441373,7.76315258636623E-7));
#15729=CARTESIAN_POINT('Ctrl Pts',(10.7389041877712,1.29777551763099,-7.54184826032082E-7));
#15730=CARTESIAN_POINT('Ctrl Pts',(10.7310976851069,1.30799836193882,-3.24039694621926E-6));
#15731=CARTESIAN_POINT('Ctrl Pts',(10.7225935645301,1.31769858917671,-8.57388820182801E-6));
#15732=CARTESIAN_POINT('Ctrl Pts',(10.7134588931078,1.3268364513864,-1.41086939541967E-5));
#15733=CARTESIAN_POINT('Ctrl Pts',(10.7004433550849,1.33985653580309,-2.19949628070403E-5));
#15734=CARTESIAN_POINT('Ctrl Pts',(10.6862650266646,1.35162127070648,-3.0022236679635E-5));
#15735=CARTESIAN_POINT('Ctrl Pts',(10.6711476119081,1.36204513612776,-3.40981369893719E-5));
#15736=CARTESIAN_POINT('Ctrl Pts',(10.6560301971515,1.37246900154903,-3.81740372991087E-5));
#15737=CARTESIAN_POINT('Ctrl Pts',(10.6399721826852,1.38155285075117,-3.83332859284948E-5));
#15738=CARTESIAN_POINT('Ctrl Pts',(10.6231652498763,1.38916602817047,-3.45204725343976E-5));
#15739=CARTESIAN_POINT('Ctrl Pts',(10.6063487480974,1.39678354012646,-3.07054883279539E-5));
#15740=CARTESIAN_POINT('Ctrl Pts',(10.5889271210941,1.40286310406803,-2.29928881382306E-5));
#15741=CARTESIAN_POINT('Ctrl Pts',(10.5711041279812,1.40730078588308,-1.53078138731408E-5));
#15742=CARTESIAN_POINT('Ctrl Pts',(10.5532811348684,1.41173846769814,-7.6227396080509E-6));
#15743=CARTESIAN_POINT('Ctrl Pts',(10.5350552605908,1.41453511891929,-9.16729947674095E-11));
#15744=CARTESIAN_POINT('Ctrl Pts',(10.5166159648474,1.4155315881283,2.48932818802672E-16));
#15745=CARTESIAN_POINT('',(10.8,-1.11638029377732,-1.39157997946485E-17));
#15746=CARTESIAN_POINT('',(10.8,1.4,0.));
#15747=CARTESIAN_POINT('',(10.5166159648474,-1.4155315881283,2.77555756156289E-17));
#15748=CARTESIAN_POINT('Ctrl Pts',(10.5166159648474,-1.4155315881283,-1.94289029309402E-16));
#15749=CARTESIAN_POINT('Ctrl Pts',(10.5344251606169,-1.41456917089032,1.72780596414851E-12));
#15750=CARTESIAN_POINT('Ctrl Pts',(10.5520727686739,-1.41197333457428,-2.53403886306205E-6));
#15751=CARTESIAN_POINT('Ctrl Pts',(10.5693578805681,-1.40785843881911,-4.04156906196095E-6));
#15752=CARTESIAN_POINT('Ctrl Pts',(10.5868701251756,-1.40368947182374,-5.56890876087065E-6));
#15753=CARTESIAN_POINT('Ctrl Pts',(10.604011804524,-1.39796079212135,-5.98742339745246E-6));
#15754=CARTESIAN_POINT('Ctrl Pts',(10.6205627760847,-1.39074087128671,-4.81856832951796E-6));
#15755=CARTESIAN_POINT('Ctrl Pts',(10.6234754753687,-1.38947028374636,-4.61286902618664E-6));
#15756=CARTESIAN_POINT('Ctrl Pts',(10.6263698187278,-1.38815339768352,-4.36721670635639E-6));
#15757=CARTESIAN_POINT('Ctrl Pts',(10.629244514885,-1.38679044403738,-4.09122931699412E-6));
#15758=CARTESIAN_POINT('Ctrl Pts',(10.6455827855986,-1.37904412775797,-2.5226612199239E-6));
#15759=CARTESIAN_POINT('Ctrl Pts',(10.6611432679573,-1.36988219838444,3.58605122725343E-7));
#15760=CARTESIAN_POINT('Ctrl Pts',(10.6757157985124,-1.35939560704671,7.40589063327193E-7));
#15761=CARTESIAN_POINT('Ctrl Pts',(10.6821516119741,-1.35476430808026,9.09288478831296E-7));
#15762=CARTESIAN_POINT('Ctrl Pts',(10.6883944859408,-1.34987400891586,5.44816430868337E-7));
#15763=CARTESIAN_POINT('Ctrl Pts',(10.6944246343503,-1.34472976213865,-9.14752338109426E-7));
#15764=CARTESIAN_POINT('Ctrl Pts',(10.7041966733629,-1.33639335368171,-3.28002794718031E-6));
#15765=CARTESIAN_POINT('Ctrl Pts',(10.7134106653983,-1.3273903805878,-8.47259327327479E-6));
#15766=CARTESIAN_POINT('Ctrl Pts',(10.7220307555455,-1.31778973409553,-1.38734771921913E-5));
#15767=CARTESIAN_POINT('Ctrl Pts',(10.7343338492722,-1.3040871333553,-2.15819326638919E-5));
#15768=CARTESIAN_POINT('Ctrl Pts',(10.7453199276401,-1.28929041974124,-2.94555326738194E-5));
#15769=CARTESIAN_POINT('Ctrl Pts',(10.7549158277293,-1.27362793268665,-3.3443536645081E-5));
#15770=CARTESIAN_POINT('Ctrl Pts',(10.7645117278185,-1.25796544563206,-3.74315406163426E-5));
#15771=CARTESIAN_POINT('Ctrl Pts',(10.7727182208071,-1.24143562566754,-3.75750290962259E-5));
#15772=CARTESIAN_POINT('Ctrl Pts',(10.7794153247677,-1.22423716044977,-3.38265125308188E-5));
#15773=CARTESIAN_POINT('Ctrl Pts',(10.7861166764432,-1.20702778690835,-3.00756184258222E-5));
#15774=CARTESIAN_POINT('Ctrl Pts',(10.7912490477072,-1.18929683429644,-2.25107044755726E-5));
#15775=CARTESIAN_POINT('Ctrl Pts',(10.7947196858669,-1.17125359626911,-1.49815203503087E-5));
#15776=CARTESIAN_POINT('Ctrl Pts',(10.7981903240266,-1.15321035824179,-7.45233622504479E-6));
#15777=CARTESIAN_POINT('Ctrl Pts',(10.7999999985278,-1.13485327409571,-1.17780195603766E-10));
#15778=CARTESIAN_POINT('Ctrl Pts',(10.8,-1.11638029377732,-1.38777878078145E-17));
#15779=CARTESIAN_POINT('',(0.276326924564679,-1.42224670711126,-5.55111512312578E-17));
#15780=CARTESIAN_POINT('Ctrl Pts',(10.5166159648474,-1.4155315881283,0.));
#15781=CARTESIAN_POINT('Ctrl Pts',(7.10318628475318,-1.599994843061,0.));
#15782=CARTESIAN_POINT('Ctrl Pts',(3.68975660465893,-1.68747752195839,0.));
#15783=CARTESIAN_POINT('Ctrl Pts',(0.276326924564679,-1.42224670711126,
0.));
#15784=CARTESIAN_POINT('',(-7.25311916552711E-19,-1.12356026268968,1.39157997946485E-17));
#15785=CARTESIAN_POINT('Ctrl Pts',(1.80411241501588E-16,-1.12356026268968,
-1.53523027623947E-16));
#15786=CARTESIAN_POINT('Ctrl Pts',(7.41078168374529E-10,-1.14141522098415,
-1.3067981184062E-11));
#15787=CARTESIAN_POINT('Ctrl Pts',(0.00163694718329378,-1.15920272117896,
-1.78823819589733E-6));
#15788=CARTESIAN_POINT('Ctrl Pts',(0.00481087395297265,-1.17671209893291,
-2.3181425555783E-6));
#15789=CARTESIAN_POINT('Ctrl Pts',(0.00802138847203439,-1.19442331774104,
-2.85415543927884E-6));
#15790=CARTESIAN_POINT('Ctrl Pts',(0.0128049030182357,-1.21185152247087,
-2.04128886843626E-6));
#15791=CARTESIAN_POINT('Ctrl Pts',(0.0191087770915565,-1.22877027194193,
1.71240493184593E-7));
#15792=CARTESIAN_POINT('Ctrl Pts',(0.0202201941454154,-1.23175316571065,
5.613248819379E-7));
#15793=CARTESIAN_POINT('Ctrl Pts',(0.0213789882593307,-1.23472016785247,
9.85829603970989E-7));
#15794=CARTESIAN_POINT('Ctrl Pts',(0.0225850188675993,-1.23766995297306,
1.43287414332239E-6));
#15795=CARTESIAN_POINT('Ctrl Pts',(0.0294291562303479,-1.25440977235863,
3.96981990042924E-6));
#15796=CARTESIAN_POINT('Ctrl Pts',(0.0377300686697735,-1.27044838970616,
7.55798501181421E-6));
#15797=CARTESIAN_POINT('Ctrl Pts',(0.0474121614036163,-1.28556782977674,
8.05058320302158E-6));
#15798=CARTESIAN_POINT('Ctrl Pts',(0.0511425121829324,-1.29139310088294,
8.24037316857697E-6));
#15799=CARTESIAN_POINT('Ctrl Pts',(0.0550784035723718,-1.29708174651376,
7.93435480917585E-6));
#15800=CARTESIAN_POINT('Ctrl Pts',(0.0592173503759339,-1.30262033374061,
6.74858081742264E-6));
#15801=CARTESIAN_POINT('Ctrl Pts',(0.0675201807396794,-1.31373087764993,
4.36988865960166E-6));
#15802=CARTESIAN_POINT('Ctrl Pts',(0.0766394565597649,-1.32423847988766,
-1.46587651676554E-6));
#15803=CARTESIAN_POINT('Ctrl Pts',(0.0864911062490747,-1.33409287340636,
-7.46705500292641E-6));
#15804=CARTESIAN_POINT('Ctrl Pts',(0.0992988409846585,-1.34690417528452,
-1.52689465211603E-5));
#15805=CARTESIAN_POINT('Ctrl Pts',(0.113232871116931,-1.35850278376499,
-2.31308069859054E-5));
#15806=CARTESIAN_POINT('Ctrl Pts',(0.128081622025101,-1.36880445085772,
-2.72849174168177E-5));
#15807=CARTESIAN_POINT('Ctrl Pts',(0.142447925282442,-1.37877140864598,
-3.13040575171566E-5));
#15808=CARTESIAN_POINT('Ctrl Pts',(0.157671864768995,-1.38752483454192,
-3.1899138628041E-5));
#15809=CARTESIAN_POINT('Ctrl Pts',(0.173588691395025,-1.39495074934422,
-2.90326641197332E-5));
#15810=CARTESIAN_POINT('Ctrl Pts',(0.189936400238013,-1.40257769006131,
-2.60885916756054E-5));
#15811=CARTESIAN_POINT('Ctrl Pts',(0.206881864105471,-1.40874232120582,
-1.95409011442111E-5));
#15812=CARTESIAN_POINT('Ctrl Pts',(0.22423558959196,-1.41334558507228,-1.29462590315495E-5));
#15813=CARTESIAN_POINT('Ctrl Pts',(0.241260467995769,-1.4178616186841,-6.47658310103417E-6));
#15814=CARTESIAN_POINT('Ctrl Pts',(0.258679581942429,-1.42087546890512,
-1.12101563992788E-10));
#15815=CARTESIAN_POINT('Ctrl Pts',(0.27632692456468,-1.42224670711126,1.05818132034585E-16));
#15816=CARTESIAN_POINT('',(0.,-1.4,0.));
#15817=CARTESIAN_POINT('',(0.292382661757373,-1.22257596919059,0.));
#15818=CARTESIAN_POINT('Ctrl Pts',(0.200274469199584,-1.12301388185427,
-2.68882138776405E-17));
#15819=CARTESIAN_POINT('Ctrl Pts',(0.200274469314753,-1.13095194822878,
-2.85686379674833E-12));
#15820=CARTESIAN_POINT('Ctrl Pts',(0.201244085522878,-1.13884856843413,
-1.08105759021766E-6));
#15821=CARTESIAN_POINT('Ctrl Pts',(0.203110344361254,-1.14653799330522,
-1.10782444979703E-6));
#15822=CARTESIAN_POINT('Ctrl Pts',(0.204308287281872,-1.15147379958167,
-1.12500597321754E-6));
#15823=CARTESIAN_POINT('Ctrl Pts',(0.205876831658669,-1.15632444796435,
-7.573778542164E-7));
#15824=CARTESIAN_POINT('Ctrl Pts',(0.207807574899602,-1.16104329283393,
-1.57887042599725E-7));
#15825=CARTESIAN_POINT('Ctrl Pts',(0.21096922807971,-1.1687705506961,8.23798139982571E-7));
#15826=CARTESIAN_POINT('Ctrl Pts',(0.215060220496011,-1.17605061753432,
2.67511715935828E-6));
#15827=CARTESIAN_POINT('Ctrl Pts',(0.220020901709485,-1.18268777995331,
1.20301732358232E-6));
#15828=CARTESIAN_POINT('Ctrl Pts',(0.222788929945646,-1.18639127392786,
3.81595076007225E-7));
#15829=CARTESIAN_POINT('Ctrl Pts',(0.225828882930032,-1.18989419630164,
-1.55522758636672E-6));
#15830=CARTESIAN_POINT('Ctrl Pts',(0.229112809647272,-1.19317965616817,
-3.52099818518546E-6));
#15831=CARTESIAN_POINT('Ctrl Pts',(0.234731790749985,-1.1988012605745,-6.88454091865859E-6));
#15832=CARTESIAN_POINT('Ctrl Pts',(0.240999377733319,-1.20372479786492,
-1.00686973618824E-5));
#15833=CARTESIAN_POINT('Ctrl Pts',(0.247759525934523,-1.2078808899968,-1.07387199666626E-5));
#15834=CARTESIAN_POINT('Ctrl Pts',(0.251104201987095,-1.20993717358883,
-1.10702228411842E-5));
#15835=CARTESIAN_POINT('Ctrl Pts',(0.254570062984725,-1.21180502729412,
-1.08478245319173E-5));
#15836=CARTESIAN_POINT('Ctrl Pts',(0.258140701417296,-1.21347208138814,
-1.01264154182862E-5));
#15837=CARTESIAN_POINT('Ctrl Pts',(0.265309933881728,-1.21681924144269,
-8.67794906268977E-6));
#15838=CARTESIAN_POINT('Ctrl Pts',(0.27282354441991,-1.21932394229889,-5.03816435877804E-6));
#15839=CARTESIAN_POINT('Ctrl Pts',(0.280540402387729,-1.22090470300999,
-2.38011023443526E-6));
#15840=CARTESIAN_POINT('Ctrl Pts',(0.284441227387562,-1.22170376798259,
-1.03647996128718E-6));
#15841=CARTESIAN_POINT('Ctrl Pts',(0.288394358015454,-1.22226603782358,
-8.41267709508591E-12));
#15842=CARTESIAN_POINT('Ctrl Pts',(0.292382661757373,-1.22257596919059,
3.10081821330854E-17));
#15843=CARTESIAN_POINT('',(0.9,-1.266106713614,0.));
#15844=CARTESIAN_POINT('Ctrl Pts',(0.29238266175737,-1.22257596919059,3.4274341177698E-16));
#15845=CARTESIAN_POINT('Ctrl Pts',(0.494894519961671,-1.23831317320793,
3.6654050078524E-12));
#15846=CARTESIAN_POINT('Ctrl Pts',(0.697432753591781,-1.25280566766171,
-2.10377631034678E-8));
#15847=CARTESIAN_POINT('Ctrl Pts',(0.900000000000002,-1.266106713614,4.80511808774455E-17));
#15848=CARTESIAN_POINT('',(0.9,1.34328341716202,0.));
#15849=CARTESIAN_POINT('',(3.5,-1.37552980833516,0.));
#15850=CARTESIAN_POINT('Ctrl Pts',(1.10000000028363,-1.27885335028943,-5.13283219638443E-11));
#15851=CARTESIAN_POINT('Ctrl Pts',(1.8994825293422,-1.32827224294784,2.51289069808066E-7));
#15852=CARTESIAN_POINT('Ctrl Pts',(2.69943073922525,-1.35940904940056,2.35357980118634E-7));
#15853=CARTESIAN_POINT('Ctrl Pts',(3.50000000097418,-1.37552980835478,8.59034485311056E-16));
#15854=CARTESIAN_POINT('',(3.5,1.44777777777778,0.));
#15855=CARTESIAN_POINT('',(7.1,-1.35793097395724,0.));
#15856=CARTESIAN_POINT('Ctrl Pts',(3.700000000362,-1.379246395385,-6.25385501848083E-12));
#15857=CARTESIAN_POINT('Ctrl Pts',(4.26467016042339,-1.38886773733237,1.63880713394601E-8));
#15858=CARTESIAN_POINT('Ctrl Pts',(4.82965558050887,-1.39115503781354,-4.12727732537403E-8));
#15859=CARTESIAN_POINT('Ctrl Pts',(5.39500817395676,-1.38725486475042,-3.97626883737645E-8));
#15860=CARTESIAN_POINT('Ctrl Pts',(5.96336684492344,-1.38333395379258,-3.82445741104923E-8));
#15861=CARTESIAN_POINT('Ctrl Pts',(6.53173538886785,-1.37316170188981,3.71969681223073E-9));
#15862=CARTESIAN_POINT('Ctrl Pts',(7.1000000000396,-1.35793097389613,-4.88946831112289E-12));
#15863=CARTESIAN_POINT('',(7.1,1.42555555555556,0.));
#15864=CARTESIAN_POINT('',(10.2,-1.23178301601145,0.));
#15865=CARTESIAN_POINT('',(10.5052647440597,-1.21555035534119,0.));
#15866=CARTESIAN_POINT('Ctrl Pts',(10.2,-1.23178301601145,-4.56855690431079E-17));
#15867=CARTESIAN_POINT('Ctrl Pts',(10.3017652114452,-1.22646242153193,-6.28718440835499E-11));
#15868=CARTESIAN_POINT('Ctrl Pts',(10.4035203469111,-1.22104923788321,1.43982679105611E-13));
#15869=CARTESIAN_POINT('Ctrl Pts',(10.5052647440597,-1.21555035534119,6.44897004721534E-17));
#15870=CARTESIAN_POINT('',(10.5997255308004,-1.11583328740478,1.38777878078145E-17));
#15871=CARTESIAN_POINT('Ctrl Pts',(10.5052647440597,-1.21555035534119,-1.86482773667507E-17));
#15872=CARTESIAN_POINT('Ctrl Pts',(10.5131888530666,-1.21512208850275,-5.60416335832109E-13));
#15873=CARTESIAN_POINT('Ctrl Pts',(10.5210180054001,-1.21372544600509,-1.35972994235015E-6));
#15874=CARTESIAN_POINT('Ctrl Pts',(10.5285917824072,-1.2114444991589,-1.66070161277884E-6));
#15875=CARTESIAN_POINT('Ctrl Pts',(10.5334522234388,-1.20998071066451,-1.8538489757029E-6));
#15876=CARTESIAN_POINT('Ctrl Pts',(10.538207639053,-1.20815156029678,-1.66445033219183E-6));
#15877=CARTESIAN_POINT('Ctrl Pts',(10.542812250732,-1.20596855068549,-1.19054254011085E-6));
#15878=CARTESIAN_POINT('Ctrl Pts',(10.5499808226381,-1.20256998801374,-4.52751316616249E-7));
#15879=CARTESIAN_POINT('Ctrl Pts',(10.5567010840309,-1.19835579238971,1.16775294480959E-6));
#15880=CARTESIAN_POINT('Ctrl Pts',(10.5628099082467,-1.1933896765605,3.12218506849373E-7));
#15881=CARTESIAN_POINT('Ctrl Pts',(10.563392699667,-1.1929159013142,2.30599178383296E-7));
#15882=CARTESIAN_POINT('Ctrl Pts',(10.563969906567,-1.19243524850296,1.23643260424227E-7));
#15883=CARTESIAN_POINT('Ctrl Pts',(10.5645413730323,-1.19194775268147,-1.33988689923433E-8));
#15884=CARTESIAN_POINT('Ctrl Pts',(10.5677990734116,-1.18916873515523,-7.94620907596477E-7));
#15885=CARTESIAN_POINT('Ctrl Pts',(10.5708705204042,-1.18616755700159,-2.52696578471864E-6));
#15886=CARTESIAN_POINT('Ctrl Pts',(10.5737438185805,-1.18296717200411,-4.3349897000341E-6));
#15887=CARTESIAN_POINT('Ctrl Pts',(10.579054042416,-1.17705244973962,-7.67644996655303E-6));
#15888=CARTESIAN_POINT('Ctrl Pts',(10.5836289246435,-1.17052745137283,-1.0999028846932E-5));
#15889=CARTESIAN_POINT('Ctrl Pts',(10.5874112735695,-1.16355342251842,-1.18035167459916E-5));
#15890=CARTESIAN_POINT('Ctrl Pts',(10.5894705469099,-1.15975646143,-1.22415145393192E-5));
#15891=CARTESIAN_POINT('Ctrl Pts',(10.5912942421259,-1.15582570378367,-1.20038889321768E-5));
#15892=CARTESIAN_POINT('Ctrl Pts',(10.5928674986933,-1.15178403025788,-1.11465830745351E-5));
#15893=CARTESIAN_POINT('Ctrl Pts',(10.5957384082276,-1.14440870489779,-9.58215448007377E-6));
#15894=CARTESIAN_POINT('Ctrl Pts',(10.5977463817932,-1.13674651935037,-5.80208140981121E-6));
#15895=CARTESIAN_POINT('Ctrl Pts',(10.5988207707371,-1.12894377506163,-2.8960211281105E-6));
#15896=CARTESIAN_POINT('Ctrl Pts',(10.5994175893465,-1.12460938291963,-1.28171667533415E-6));
#15897=CARTESIAN_POINT('Ctrl Pts',(10.5997255306822,-1.12023121224821,-9.4020583932734E-12));
#15898=CARTESIAN_POINT('Ctrl Pts',(10.5997255308004,-1.11583328740478,-9.97465998686664E-18));
#15899=CARTESIAN_POINT('',(10.5997255308004,1.11583328740478,0.));
#15900=CARTESIAN_POINT('',(10.5997255308004,0.7,0.));
#15901=CARTESIAN_POINT('',(10.5052647440597,1.21555035534119,0.));
#15902=CARTESIAN_POINT('Ctrl Pts',(10.5997255308004,1.11583328740478,8.8037216405823E-17));
#15903=CARTESIAN_POINT('Ctrl Pts',(10.5997255307124,1.12376989384288,-2.22024716398596E-12));
#15904=CARTESIAN_POINT('Ctrl Pts',(10.5987536115518,1.13166401228391,-1.27532141444775E-6));
#15905=CARTESIAN_POINT('Ctrl Pts',(10.5968849989732,1.13935090273995,-1.5236651967046E-6));
#15906=CARTESIAN_POINT('Ctrl Pts',(10.5956849616024,1.14428748291596,-1.68315348385219E-6));
#15907=CARTESIAN_POINT('Ctrl Pts',(10.5941139374364,1.14913880701507,-1.46899737395989E-6));
#15908=CARTESIAN_POINT('Ctrl Pts',(10.5921809408638,1.1538584293407,-9.90118991603547E-7));
#15909=CARTESIAN_POINT('Ctrl Pts',(10.5891742477341,1.16119959911942,-2.45244239835432E-7));
#15910=CARTESIAN_POINT('Ctrl Pts',(10.5853292249979,1.16813727090899,1.33309554558619E-6));
#15911=CARTESIAN_POINT('Ctrl Pts',(10.5807005079991,1.17450509276749,4.08358240744415E-7));
#15912=CARTESIAN_POINT('Ctrl Pts',(10.5802604812716,1.17511044665166,3.20448539159982E-7));
#15913=CARTESIAN_POINT('Ctrl Pts',(10.5798133373602,1.17571063303672,2.07176952714776E-7));
#15914=CARTESIAN_POINT('Ctrl Pts',(10.5793591019426,1.17630549598644,6.38823567561716E-8));
#15915=CARTESIAN_POINT('Ctrl Pts',(10.5767566952267,1.17971358631841,-7.57081408668461E-7));
#15916=CARTESIAN_POINT('Ctrl Pts',(10.5739217504488,1.18294722379721,-2.53660858190298E-6));
#15917=CARTESIAN_POINT('Ctrl Pts',(10.570876618072,1.18599321478588,-4.38998728286835E-6));
#15918=CARTESIAN_POINT('Ctrl Pts',(10.5652565693637,1.19161484813492,-7.81055403847458E-6));
#15919=CARTESIAN_POINT('Ctrl Pts',(10.5589874561388,1.19653507038546,-1.11999964534866E-5));
#15920=CARTESIAN_POINT('Ctrl Pts',(10.5522271124844,1.20068789486255,-1.20263298844839E-5));
#15921=CARTESIAN_POINT('Ctrl Pts',(10.5485500617744,1.20294667739977,-1.24757848359648E-5));
#15922=CARTESIAN_POINT('Ctrl Pts',(10.5447269560479,1.20497781184918,-1.22374322375965E-5));
#15923=CARTESIAN_POINT('Ctrl Pts',(10.5407797717187,1.20676523914267,-1.13674773191707E-5));
#15924=CARTESIAN_POINT('Ctrl Pts',(10.5335711832013,1.210029547771,-9.77871264224002E-6));
#15925=CARTESIAN_POINT('Ctrl Pts',(10.5260296312848,1.21244761587922,-5.9245235663186E-6));
#15926=CARTESIAN_POINT('Ctrl Pts',(10.5182973307397,1.21394093281975,-2.95733858081469E-6));
#15927=CARTESIAN_POINT('Ctrl Pts',(10.514004731837,1.21476995008607,-1.31010113336685E-6));
#15928=CARTESIAN_POINT('Ctrl Pts',(10.5096528988527,1.21531319279956,-7.28166367327128E-12));
#15929=CARTESIAN_POINT('Ctrl Pts',(10.5052647440597,1.21555035534119,-3.31765864780564E-17));
#15930=CARTESIAN_POINT('',(10.2,1.23178301601145,0.));
#15931=CARTESIAN_POINT('Ctrl Pts',(10.5052647440597,1.21555035534119,1.20285454773689E-16));
#15932=CARTESIAN_POINT('Ctrl Pts',(10.4035203468995,1.22104923788384,1.44021921739714E-13));
#15933=CARTESIAN_POINT('Ctrl Pts',(10.3017652114309,1.22646242153268,-6.28696045710378E-11));
#15934=CARTESIAN_POINT('Ctrl Pts',(10.2,1.23178301601145,1.23125603768043E-16));
#15935=CARTESIAN_POINT('',(10.2,-1.30754691548544,0.));
#15936=CARTESIAN_POINT('Origin',(8.8,0.,0.));
#15937=CARTESIAN_POINT('',(8.4,-4.89858719658942E-17,0.));
#15938=CARTESIAN_POINT('Origin',(2.,0.,0.));
#15939=CARTESIAN_POINT('',(1.6,-4.89858719658941E-17,0.7));
#15940=CARTESIAN_POINT('Origin',(2.,0.,0.7));
#15941=CARTESIAN_POINT('',(1.6,-4.89858719658941E-17,0.));
#15942=CARTESIAN_POINT('Origin',(10.2,-1.30754691548544,0.));
#15943=CARTESIAN_POINT('',(10.1999999975107,-1.19856231453552,0.605472757505173));
#15944=CARTESIAN_POINT('Ctrl Pts',(10.2,-1.23178301601145,0.));
#15945=CARTESIAN_POINT('Ctrl Pts',(10.2,-1.22625045235593,0.100869147801815));
#15946=CARTESIAN_POINT('Ctrl Pts',(10.2,-1.22071692450357,0.201739022585575));
#15947=CARTESIAN_POINT('Ctrl Pts',(10.2,-1.2096433936729,0.403562754186249));
#15948=CARTESIAN_POINT('Ctrl Pts',(10.1999999975107,-1.20410330368611,0.50451817268257));
#15949=CARTESIAN_POINT('Ctrl Pts',(10.1999999975107,-1.19856231453552,0.605472757505173));
#15950=CARTESIAN_POINT('',(10.1999999975107,1.19856231453552,0.605472757505173));
#15951=CARTESIAN_POINT('Ctrl Pts',(10.1999999975107,1.19856231453552,0.605472757505173));
#15952=CARTESIAN_POINT('Ctrl Pts',(10.1999999975107,1.20410418062036,0.504502195294633));
#15953=CARTESIAN_POINT('Ctrl Pts',(10.2,1.20964514726505,0.403530798997214));
#15954=CARTESIAN_POINT('Ctrl Pts',(10.2,1.22071867750565,0.201707067365009));
#15955=CARTESIAN_POINT('Ctrl Pts',(10.2,1.22625132869937,0.100853170395858));
#15956=CARTESIAN_POINT('Ctrl Pts',(10.2,1.23178301601145,0.));
#15957=CARTESIAN_POINT('',(10.1999999980542,1.09857320530976,0.7));
#15958=CARTESIAN_POINT('Ctrl Pts',(10.1999999999973,1.09857320510493,0.7));
#15959=CARTESIAN_POINT('Ctrl Pts',(10.2000000008642,1.10649088744708,0.699999999248278));
#15960=CARTESIAN_POINT('Ctrl Pts',(10.1999989363772,1.11434529358656,0.699006164779054));
#15961=CARTESIAN_POINT('Ctrl Pts',(10.1999980093114,1.12199598895487,0.697118997523365));
#15962=CARTESIAN_POINT('Ctrl Pts',(10.1999974900707,1.12628106973794,0.696062013320951));
#15963=CARTESIAN_POINT('Ctrl Pts',(10.1999970168623,1.13050229860485,0.694723760583242));
#15964=CARTESIAN_POINT('Ctrl Pts',(10.199996713894,1.13463332887353,0.693115046692397));
#15965=CARTESIAN_POINT('Ctrl Pts',(10.1999961690675,1.14206214329588,0.690222103243312));
#15966=CARTESIAN_POINT('Ctrl Pts',(10.1999962772589,1.14911941279843,0.686488866209959));
#15967=CARTESIAN_POINT('Ctrl Pts',(10.1999969599022,1.15565885618684,0.681996408643444));
#15968=CARTESIAN_POINT('Ctrl Pts',(10.1999973343062,1.15924549304116,0.679532465931891));
#15969=CARTESIAN_POINT('Ctrl Pts',(10.1999978674396,1.16267609380848,0.676839263748528));
#15970=CARTESIAN_POINT('Ctrl Pts',(10.1999983417863,1.16592263776853,0.673924718551186));
#15971=CARTESIAN_POINT('Ctrl Pts',(10.199998806773,1.16910511991263,0.671067684066867));
#15972=CARTESIAN_POINT('Ctrl Pts',(10.1999992207276,1.17209141256199,0.668015240668471));
#15973=CARTESIAN_POINT('Ctrl Pts',(10.1999992206607,1.17485880184773,0.664778864469812));
#15974=CARTESIAN_POINT('Ctrl Pts',(10.1999992205369,1.17997899231675,0.658790960038769));
#15975=CARTESIAN_POINT('Ctrl Pts',(10.1999979581638,1.18435276586188,0.652174799271591));
#15976=CARTESIAN_POINT('Ctrl Pts',(10.1999975326045,1.18791964688485,0.645095405674036));
#15977=CARTESIAN_POINT('Ctrl Pts',(10.1999974898604,1.18827791229431,0.644384335742179));
#15978=CARTESIAN_POINT('Ctrl Pts',(10.1999974535047,1.18862799840101,0.643668573506599));
#15979=CARTESIAN_POINT('Ctrl Pts',(10.1999974242393,1.18896981696374,0.64294827577739));
#15980=CARTESIAN_POINT('Ctrl Pts',(10.1999971329942,1.1923715530028,0.635779961907205));
#15981=CARTESIAN_POINT('Ctrl Pts',(10.1999977790614,1.19491900203126,0.628247233077589));
#15982=CARTESIAN_POINT('Ctrl Pts',(10.1999987199397,1.19655829940385,0.620518158911201));
#15983=CARTESIAN_POINT('Ctrl Pts',(10.1999993222661,1.19760773597399,0.615570201805241));
#15984=CARTESIAN_POINT('Ctrl Pts',(10.2,1.19828413277105,0.610541112135461));
#15985=CARTESIAN_POINT('Ctrl Pts',(10.2,1.19856231427281,0.60547275750556));
#15986=CARTESIAN_POINT('',(10.2,-1.09857320510402,0.7));
#15987=CARTESIAN_POINT('',(10.2,-0.653773457742722,0.7));
#15988=CARTESIAN_POINT('Ctrl Pts',(10.2,-1.19856231427281,0.60547275750556));
#15989=CARTESIAN_POINT('Ctrl Pts',(10.2,-1.19812809376428,0.613384079828744));
#15990=CARTESIAN_POINT('Ctrl Pts',(10.1999984889428,-1.1967261327477,0.621202329970501));
#15991=CARTESIAN_POINT('Ctrl Pts',(10.1999978161146,-1.19444079525024,0.628767398200536));
#15992=CARTESIAN_POINT('Ctrl Pts',(10.1999974438306,-1.19317629038787,0.632953241898348));
#15993=CARTESIAN_POINT('Ctrl Pts',(10.1999972759003,-1.19164034846853,0.637061602680377));
#15994=CARTESIAN_POINT('Ctrl Pts',(10.1999973648938,-1.18984073583679,0.641063423920242));
#15995=CARTESIAN_POINT('Ctrl Pts',(10.1999975257516,-1.18658789218766,0.648296813248274));
#15996=CARTESIAN_POINT('Ctrl Pts',(10.1999986492083,-1.18251199594868,0.655103972585077));
#15997=CARTESIAN_POINT('Ctrl Pts',(10.1999990866637,-1.1776776067306,0.66132208754656));
#15998=CARTESIAN_POINT('Ctrl Pts',(10.1999991692372,-1.17676507450965,0.662495809810115));
#15999=CARTESIAN_POINT('Ctrl Pts',(10.1999992204458,-1.17582538639523,0.663648473741297));
#16000=CARTESIAN_POINT('Ctrl Pts',(10.1999992199672,-1.17485880188435,0.664778864469789));
#16001=CARTESIAN_POINT('Ctrl Pts',(10.1999992190419,-1.17299032792757,0.666963987046661));
#16002=CARTESIAN_POINT('Ctrl Pts',(10.1999990265713,-1.17102137903347,0.669065925022507));
#16003=CARTESIAN_POINT('Ctrl Pts',(10.1999987631451,-1.16895889720817,0.671081139337088));
#16004=CARTESIAN_POINT('Ctrl Pts',(10.1999980371048,-1.16327440276409,0.676635357771578));
#16005=CARTESIAN_POINT('Ctrl Pts',(10.1999968952367,-1.15694629605269,0.681471105251756));
#16006=CARTESIAN_POINT('Ctrl Pts',(10.1999965193249,-1.15013861030111,0.685534582868085));
#16007=CARTESIAN_POINT('Ctrl Pts',(10.1999962798276,-1.14580136285465,0.688123466749966));
#16008=CARTESIAN_POINT('Ctrl Pts',(10.1999963003895,-1.14126848503633,0.690398200126003));
#16009=CARTESIAN_POINT('Ctrl Pts',(10.1999965837416,-1.13657664085124,0.692335536714198));
#16010=CARTESIAN_POINT('Ctrl Pts',(10.199997026059,-1.12925259320479,0.695359751696499));
#16011=CARTESIAN_POINT('Ctrl Pts',(10.1999981114625,-1.12162598460505,0.697529439192009));
#16012=CARTESIAN_POINT('Ctrl Pts',(10.1999989867727,-1.11384404680861,0.698775198878229));
#16013=CARTESIAN_POINT('Ctrl Pts',(10.1999995533653,-1.10880676031141,0.699581585232154));
#16014=CARTESIAN_POINT('Ctrl Pts',(10.200000000559,-1.10370379302489,0.699999999512891));
#16015=CARTESIAN_POINT('Ctrl Pts',(10.1999999999973,-1.09857320510493,0.7));
#16016=CARTESIAN_POINT('Ctrl Pts',(10.0273290644374,-1.24073895154929,-0.000342977371441382));
#16017=CARTESIAN_POINT('Ctrl Pts',(10.0182194939277,-1.2301570933055,0.201590462913323));
#16018=CARTESIAN_POINT('Ctrl Pts',(10.0091098064739,-1.21957524432673,0.403523898419685));
#16019=CARTESIAN_POINT('Ctrl Pts',(10.,-1.20899340483173,0.605457329065658));
#16020=CARTESIAN_POINT('Ctrl Pts',(9.11786336174441,-1.287320026752,-0.000205293215301774));
#16021=CARTESIAN_POINT('Ctrl Pts',(9.11054075262461,-1.27673792859995,0.201728409731728));
#16022=CARTESIAN_POINT('Ctrl Pts',(9.10321803982027,-1.2661558351744,0.403662109352091));
#16023=CARTESIAN_POINT('Ctrl Pts',(9.09589522044064,-1.25557375159922,0.605595805683776));
#16024=CARTESIAN_POINT('Ctrl Pts',(8.20875307681921,-1.32613868191631,-8.19769783003664E-5));
#16025=CARTESIAN_POINT('Ctrl Pts',(8.20321812688803,-1.31555630757271,0.201851960079368));
#16026=CARTESIAN_POINT('Ctrl Pts',(8.19768309032111,-1.30497393555236,0.403785895133155));
#16027=CARTESIAN_POINT('Ctrl Pts',(8.19214796413157,-1.29439157095064,0.605719828258773));
#16028=CARTESIAN_POINT('Ctrl Pts',(7.29999999999999,-1.35236351479115,1.04083408558608E-17));
#16029=CARTESIAN_POINT('Ctrl Pts',(7.29625341766944,-1.34178092325774,0.201934092022114));
#16030=CARTESIAN_POINT('Ctrl Pts',(7.2925067690755,-1.33119833465137,0.403868182971915));
#16031=CARTESIAN_POINT('Ctrl Pts',(7.28876005303739,-1.32061574904145,0.605802272831199));
#16032=CARTESIAN_POINT('Ctrl Pts',(7.29999999953094,-1.32031613471704,0.605285370449856));
#16033=CARTESIAN_POINT('Ctrl Pts',(8.20058408060299,-1.29406305600824,0.605326635812744));
#16034=CARTESIAN_POINT('Ctrl Pts',(9.10058974048747,-1.25534320916473,0.605388449123016));
#16035=CARTESIAN_POINT('Ctrl Pts',(9.99999999968202,-1.20899340489109,0.605457329065633));
#16036=CARTESIAN_POINT('Ctrl Pts',(10.5052670937641,-1.21555282972197,-4.72190879230918E-5));
#16037=CARTESIAN_POINT('Ctrl Pts',(10.4952228315222,-1.20497561405085,0.201799837144789));
#16038=CARTESIAN_POINT('Ctrl Pts',(10.4851784461209,-1.19439840869387,0.403646887802288));
#16039=CARTESIAN_POINT('Ctrl Pts',(10.4751339353761,-1.18382121389426,0.605493932788863));
#16040=CARTESIAN_POINT('Ctrl Pts',(10.4035069533234,-1.22105168617584,-3.13467776074076E-5));
#16041=CARTESIAN_POINT('Ctrl Pts',(10.3936624949941,-1.21047444506522,0.201815739766394));
#16042=CARTESIAN_POINT('Ctrl Pts',(10.3838179147697,-1.19989721405033,0.403662820908308));
#16043=CARTESIAN_POINT('Ctrl Pts',(10.3739732104882,-1.18931999337004,0.605509896555428));
#16044=CARTESIAN_POINT('Ctrl Pts',(10.3017512542637,-1.22646400658821,-1.55943981238903E-5));
#16045=CARTESIAN_POINT('Ctrl Pts',(10.2921066085356,-1.21588673949083,0.201831522212972));
#16046=CARTESIAN_POINT('Ctrl Pts',(10.2824618422276,-1.20530948226626,0.403678633593635));
#16047=CARTESIAN_POINT('Ctrl Pts',(10.2728169532007,-1.19473223514815,0.605525739654126));
#16048=CARTESIAN_POINT('Ctrl Pts',(10.2,-1.23178301601145,-4.5102810375397E-17));
#16049=CARTESIAN_POINT('Ctrl Pts',(10.1905551755811,-1.22120572247414,0.20184714636246));
#16050=CARTESIAN_POINT('Ctrl Pts',(10.1811102319487,-1.21062843858304,0.403694287664275));
#16051=CARTESIAN_POINT('Ctrl Pts',(10.1716651669877,-1.20005116456574,0.605541423818621));
#16052=CARTESIAN_POINT('',(10.4735630903435,-1.18390659316268,0.605494180667944));
#16053=CARTESIAN_POINT('Ctrl Pts',(10.1999999975038,-1.19856231440453,0.605472757505366));
#16054=CARTESIAN_POINT('Ctrl Pts',(10.2911933328565,-1.19375025772558,0.605479840815741));
#16055=CARTESIAN_POINT('Ctrl Pts',(10.3823809652617,-1.18886335120032,0.605486986548286));
#16056=CARTESIAN_POINT('Ctrl Pts',(10.4735630903435,-1.18390659316268,0.605494180667944));
#16057=CARTESIAN_POINT('Ctrl Pts',(10.4735630903435,-1.18390659316268,0.605494180667945));
#16058=CARTESIAN_POINT('Ctrl Pts',(10.4841302498201,-1.19445434834508,0.403662775875149));
#16059=CARTESIAN_POINT('Ctrl Pts',(10.4946974680575,-1.20500226999407,0.201831382381129));
#16060=CARTESIAN_POINT('Ctrl Pts',(10.5052647440597,-1.21555035534119,-6.86299975183324E-17));
#16061=CARTESIAN_POINT('Ctrl Pts',(10.,-1.10900986674273,0.7));
#16062=CARTESIAN_POINT('Ctrl Pts',(9.09944331332257,-1.15544418981837,0.7));
#16063=CARTESIAN_POINT('Ctrl Pts',(8.1984670949788,-1.19422430779862,0.7));
#16064=CARTESIAN_POINT('Ctrl Pts',(7.29709043526679,-1.22049830417059,0.7));
#16065=CARTESIAN_POINT('Ctrl Pts',(10.0014871213396,-1.13785139984992,0.7));
#16066=CARTESIAN_POINT('Ctrl Pts',(9.10076698492608,-1.18430758604571,0.700000491839571));
#16067=CARTESIAN_POINT('Ctrl Pts',(8.19957769811723,-1.22310890030201,0.699999704549177));
#16068=CARTESIAN_POINT('Ctrl Pts',(7.29793284700475,-1.24939875264889,0.7));
#16069=CARTESIAN_POINT('Ctrl Pts',(10.0040646682326,-1.18784086746588,0.676686753673613));
#16070=CARTESIAN_POINT('Ctrl Pts',(9.10306300621911,-1.23433322993607,0.676664155483858));
#16071=CARTESIAN_POINT('Ctrl Pts',(8.20149954052229,-1.27317186922949,0.676644146017133));
#16072=CARTESIAN_POINT('Ctrl Pts',(7.29939288958795,-1.29948813715084,0.676630595533454));
#16073=CARTESIAN_POINT('Ctrl Pts',(10.0050807923581,-1.20754778500352,0.627085325222079));
#16074=CARTESIAN_POINT('Ctrl Pts',(9.10396596140607,-1.25402923300358,0.627026849623412));
#16075=CARTESIAN_POINT('Ctrl Pts',(8.20225661204673,-1.29285896783792,0.626974637782525));
#16076=CARTESIAN_POINT('Ctrl Pts',(7.29996660609514,-1.31917051289423,0.626939603849942));
#16077=CARTESIAN_POINT('Ctrl Pts',(10.0051416645797,-1.20872835322339,0.605457722909465));
#16078=CARTESIAN_POINT('Ctrl Pts',(9.1040197884667,-1.25519559703033,0.605388684776982));
#16079=CARTESIAN_POINT('Ctrl Pts',(8.20230020786566,-1.29401302889245,0.605326714446839));
#16080=CARTESIAN_POINT('Ctrl Pts',(7.29999999953094,-1.32031613471704,0.605285370449856));
#16081=CARTESIAN_POINT('Ctrl Pts',(10.4681436286308,-1.08420482079362,0.7));
#16082=CARTESIAN_POINT('Ctrl Pts',(10.3770124662346,-1.0891584122264,0.7));
#16083=CARTESIAN_POINT('Ctrl Pts',(10.285877616441,-1.09404209584202,0.7));
#16084=CARTESIAN_POINT('Ctrl Pts',(10.1947388861048,-1.09885088260188,0.7));
#16085=CARTESIAN_POINT('Ctrl Pts',(10.4697107510168,-1.11303515260326,0.7));
#16086=CARTESIAN_POINT('Ctrl Pts',(10.3785648662465,-1.11799094453753,0.700000051218742));
#16087=CARTESIAN_POINT('Ctrl Pts',(10.2874149314686,-1.12287675076168,0.699999949550842));
#16088=CARTESIAN_POINT('Ctrl Pts',(10.196260416419,-1.12768774893097,0.7));
#16089=CARTESIAN_POINT('Ctrl Pts',(10.4724269697127,-1.16300539549315,0.676698381019543));
#16090=CARTESIAN_POINT('Ctrl Pts',(10.3812557252598,-1.16796482352885,0.676696026813929));
#16091=CARTESIAN_POINT('Ctrl Pts',(10.2900793016129,-1.17285439035486,0.676693724638983));
#16092=CARTESIAN_POINT('Ctrl Pts',(10.1988975981852,-1.17766904563614,0.67669140632491));
#16093=CARTESIAN_POINT('Ctrl Pts',(10.4734985149421,-1.18271860027509,0.627116141711795));
#16094=CARTESIAN_POINT('Ctrl Pts',(10.382317043787,-1.18767684023183,0.627110048826767));
#16095=CARTESIAN_POINT('Ctrl Pts',(10.2911301919381,-1.19256517083271,0.627104033151799));
#16096=CARTESIAN_POINT('Ctrl Pts',(10.1999375452555,-1.19737868557977,0.627098033786781));
#16097=CARTESIAN_POINT('Ctrl Pts',(10.4735630903435,-1.18390659316268,0.605494180667944));
#16098=CARTESIAN_POINT('Ctrl Pts',(10.3823809652617,-1.18886335120032,0.605486986548286));
#16099=CARTESIAN_POINT('Ctrl Pts',(10.2911933328565,-1.19375025772558,0.605479840815741));
#16100=CARTESIAN_POINT('Ctrl Pts',(10.1999999975038,-1.19856231440453,0.605472757505366));
#16101=CARTESIAN_POINT('',(10.4681436258201,-1.08420482094639,0.7));
#16102=CARTESIAN_POINT('Ctrl Pts',(10.4681436258201,-1.0842048209464,0.7));
#16103=CARTESIAN_POINT('Ctrl Pts',(10.3787660248044,-1.08906309452597,0.7));
#16104=CARTESIAN_POINT('Ctrl Pts',(10.289384876933,-1.09385412476048,0.7));
#16105=CARTESIAN_POINT('Ctrl Pts',(10.1999999999973,-1.09857320510493,0.7));
#16106=CARTESIAN_POINT('Origin',(10.4681436286308,-1.08420482099672,0.6));
#16107=CARTESIAN_POINT('Origin',(5.4,-8.11656130105013E-18,0.7));
#16108=CARTESIAN_POINT('',(10.4681436286308,1.08420482109828,0.7));
#16109=CARTESIAN_POINT('Ctrl Pts',(10.1999999980461,1.09857320520795,0.7));
#16110=CARTESIAN_POINT('Ctrl Pts',(10.2893848765692,1.09385412478074,0.7));
#16111=CARTESIAN_POINT('Ctrl Pts',(10.3787660260279,1.08906309446088,0.7));
#16112=CARTESIAN_POINT('Ctrl Pts',(10.4681436286308,1.08420482079361,0.7));
#16113=CARTESIAN_POINT('',(10.4681436286308,0.7,0.7));
#16114=CARTESIAN_POINT('Ctrl Pts',(7.3,1.35236351479305,-3.57463069561303E-11));
#16115=CARTESIAN_POINT('Ctrl Pts',(7.29625341766908,1.34178092325856,0.20193409200674));
#16116=CARTESIAN_POINT('Ctrl Pts',(7.29250676907475,1.33119833465113,0.403868182976914));
#16117=CARTESIAN_POINT('Ctrl Pts',(7.28876005303626,1.32061574904014,0.60580227285657));
#16118=CARTESIAN_POINT('Ctrl Pts',(8.20875307682014,1.32613868191819,-8.19770140467192E-5));
#16119=CARTESIAN_POINT('Ctrl Pts',(8.20321812688841,1.31555630757352,0.201851960063995));
#16120=CARTESIAN_POINT('Ctrl Pts',(8.19768309032092,1.3049739355521,0.403785895138154));
#16121=CARTESIAN_POINT('Ctrl Pts',(8.19214796413082,1.29439157094932,0.605719828284144));
#16122=CARTESIAN_POINT('Ctrl Pts',(9.11786336174626,1.28732002675385,-0.000205293251048056));
#16123=CARTESIAN_POINT('Ctrl Pts',(9.11054075262572,1.27673792860073,0.201728409716354));
#16124=CARTESIAN_POINT('Ctrl Pts',(9.10321803982063,1.26615583517412,0.403662109357089));
#16125=CARTESIAN_POINT('Ctrl Pts',(9.09589522044026,1.25557375159787,0.605595805709147));
#16126=CARTESIAN_POINT('Ctrl Pts',(10.0273290644402,1.2407389515511,-0.000342977407187712));
#16127=CARTESIAN_POINT('Ctrl Pts',(10.0182194939295,1.23015709330624,0.201590462897949));
#16128=CARTESIAN_POINT('Ctrl Pts',(10.0091098064748,1.21957524432641,0.403523898424684));
#16129=CARTESIAN_POINT('Ctrl Pts',(10.,1.20899340483035,0.605457329091028));
#16130=CARTESIAN_POINT('Ctrl Pts',(10.2,1.23178301601276,-2.39624899783797E-11));
#16131=CARTESIAN_POINT('Ctrl Pts',(10.1905551755807,1.22120572247504,0.201847146346486));
#16132=CARTESIAN_POINT('Ctrl Pts',(10.1811102319479,1.21062843858352,0.403694287656288));
#16133=CARTESIAN_POINT('Ctrl Pts',(10.1716651669865,1.2000511645658,0.605541423818621));
#16134=CARTESIAN_POINT('Ctrl Pts',(10.3017512542641,1.22646400658951,-1.55944220863836E-5));
#16135=CARTESIAN_POINT('Ctrl Pts',(10.2921066085356,1.2158867394917,0.201831522196997));
#16136=CARTESIAN_POINT('Ctrl Pts',(10.2824618422272,1.20530948226672,0.403678633585648));
#16137=CARTESIAN_POINT('Ctrl Pts',(10.2728169531999,1.19473223514819,0.605525739654127));
#16138=CARTESIAN_POINT('Ctrl Pts',(10.4035069533242,1.22105168617711,-3.13468015701665E-5));
#16139=CARTESIAN_POINT('Ctrl Pts',(10.3936624949945,1.21047444506608,0.201815739750419));
#16140=CARTESIAN_POINT('Ctrl Pts',(10.3838179147698,1.19989721405077,0.40366282090032));
#16141=CARTESIAN_POINT('Ctrl Pts',(10.3739732104878,1.18931999337006,0.605509896555428));
#16142=CARTESIAN_POINT('Ctrl Pts',(10.5052670937653,1.21555282972323,-4.72191118859062E-5));
#16143=CARTESIAN_POINT('Ctrl Pts',(10.495222831523,1.20497561405169,0.201799837128814));
#16144=CARTESIAN_POINT('Ctrl Pts',(10.4851784461213,1.19439840869429,0.403646887794301));
#16145=CARTESIAN_POINT('Ctrl Pts',(10.4751339353761,1.18382121389426,0.605493932788864));
#16146=CARTESIAN_POINT('',(10.4735630903435,1.18390659316268,0.605494180667944));
#16147=CARTESIAN_POINT('Ctrl Pts',(10.5052647440597,1.21555035534119,-4.0462425077159E-16));
#16148=CARTESIAN_POINT('Ctrl Pts',(10.4946974680575,1.20500226999407,0.201831382381129));
#16149=CARTESIAN_POINT('Ctrl Pts',(10.4841302498201,1.19445434834508,0.40366277587515));
#16150=CARTESIAN_POINT('Ctrl Pts',(10.4735630903435,1.18390659316268,0.605494180667945));
#16151=CARTESIAN_POINT('Ctrl Pts',(10.4735630903435,1.18390659316268,0.605494180667944));
#16152=CARTESIAN_POINT('Ctrl Pts',(10.3823809652617,1.18886335120032,0.605486986548286));
#16153=CARTESIAN_POINT('Ctrl Pts',(10.2911933328565,1.19375025772558,0.605479840815741));
#16154=CARTESIAN_POINT('Ctrl Pts',(10.1999999975038,1.19856231440453,0.605472757505366));
#16155=CARTESIAN_POINT('Origin',(7.1,1.42555555555556,0.));
#16156=CARTESIAN_POINT('',(7.0999999994629,-1.32593912634735,0.605276549957215));
#16157=CARTESIAN_POINT('Ctrl Pts',(7.0999999994629,-1.32593912634735,0.605276549957215));
#16158=CARTESIAN_POINT('Ctrl Pts',(7.0999999994629,-1.33126650931098,0.504490734647167));
#16159=CARTESIAN_POINT('Ctrl Pts',(7.1,-1.33659376385849,0.403703958452373));
#16160=CARTESIAN_POINT('Ctrl Pts',(7.1,-1.3472576786761,0.201945747207886));
#16161=CARTESIAN_POINT('Ctrl Pts',(7.1,-1.35259443928223,0.100972400854069));
#16162=CARTESIAN_POINT('Ctrl Pts',(7.1,-1.35793097395724,0.));
#16163=CARTESIAN_POINT('',(7.1,-1.22604182196417,0.7));
#16164=CARTESIAN_POINT('Ctrl Pts',(7.1,-1.22604182196307,0.7));
#16165=CARTESIAN_POINT('Ctrl Pts',(7.1,-1.23395163718705,0.7));
#16166=CARTESIAN_POINT('Ctrl Pts',(7.09999945440688,-1.24179783218049,0.699006056038995));
#16167=CARTESIAN_POINT('Ctrl Pts',(7.09999897931553,-1.2494401870438,0.697119011207626));
#16168=CARTESIAN_POINT('Ctrl Pts',(7.09999871186578,-1.25374240366384,0.696056710937424));
#16169=CARTESIAN_POINT('Ctrl Pts',(7.09999846845149,-1.25798007942473,0.69471034534287));
#16170=CARTESIAN_POINT('Ctrl Pts',(7.09999831430822,-1.26212651101681,0.6930909329195));
#16171=CARTESIAN_POINT('Ctrl Pts',(7.09999803835695,-1.26954956016987,0.690191818885951));
#16172=CARTESIAN_POINT('Ctrl Pts',(7.09999810102228,-1.27659977900265,0.686452252582521));
#16173=CARTESIAN_POINT('Ctrl Pts',(7.09999845706054,-1.28313109767173,0.681953977461377));
#16174=CARTESIAN_POINT('Ctrl Pts',(7.09999865314126,-1.2867280867584,0.679476645189077));
#16175=CARTESIAN_POINT('Ctrl Pts',(7.09999893113315,-1.29016742765117,0.67676830886676));
#16176=CARTESIAN_POINT('Ctrl Pts',(7.09999917787259,-1.2934208019838,0.673837071833988));
#16177=CARTESIAN_POINT('Ctrl Pts',(7.09999941835505,-1.29659167515528,0.670980166997299));
#16178=CARTESIAN_POINT('Ctrl Pts',(7.09999963169439,-1.29956664557352,0.667928795646746));
#16179=CARTESIAN_POINT('Ctrl Pts',(7.09999963110542,-1.30232317314677,0.664694459428825));
#16180=CARTESIAN_POINT('Ctrl Pts',(7.09999963001387,-1.30743194453681,0.658700148145236));
#16181=CARTESIAN_POINT('Ctrl Pts',(7.09999897381858,-1.31179333085743,0.652078782729069));
#16182=CARTESIAN_POINT('Ctrl Pts',(7.09999874753952,-1.31534789998199,0.64499600756552));
#16183=CARTESIAN_POINT('Ctrl Pts',(7.09999872438549,-1.31571162172319,0.644271261689237));
#16184=CARTESIAN_POINT('Ctrl Pts',(7.0999987046402,-1.31606685549941,0.643541664816448));
#16185=CARTESIAN_POINT('Ctrl Pts',(7.09999868869212,-1.31641350913238,0.642807383257706));
#16186=CARTESIAN_POINT('Ctrl Pts',(7.09999853283271,-1.31980133087414,0.635631300872562));
#16187=CARTESIAN_POINT('Ctrl Pts',(7.09999885939544,-1.32233451509485,0.628092322434426));
#16188=CARTESIAN_POINT('Ctrl Pts',(7.09999934101855,-1.32395982399511,0.620358959365968));
#16189=CARTESIAN_POINT('Ctrl Pts',(7.09999964997549,-1.32500244522074,0.615398075635307));
#16190=CARTESIAN_POINT('Ctrl Pts',(7.09999999934316,-1.32567060646853,0.610356529630438));
#16191=CARTESIAN_POINT('Ctrl Pts',(7.09999999981141,-1.32593912630714,0.60527654995744));
#16192=CARTESIAN_POINT('',(7.09999999995537,1.22604182196549,0.7));
#16193=CARTESIAN_POINT('',(7.1,0.712777777777778,0.7));
#16194=CARTESIAN_POINT('',(7.0999999994629,1.32593912634735,0.605276549957215));
#16195=CARTESIAN_POINT('Ctrl Pts',(7.09999999981142,1.32593912630714,0.60527654995744));
#16196=CARTESIAN_POINT('Ctrl Pts',(7.09999999908198,1.32552083177145,0.613190035045322));
#16197=CARTESIAN_POINT('Ctrl Pts',(7.09999922367565,1.32413525001942,0.621012727860624));
#16198=CARTESIAN_POINT('Ctrl Pts',(7.09999888117586,1.32186630199077,0.628584136488803));
#16199=CARTESIAN_POINT('Ctrl Pts',(7.09999868987568,1.32059900146923,0.632813078704371));
#16200=CARTESIAN_POINT('Ctrl Pts',(7.09999860640034,1.3190551184949,0.636963663611311));
#16201=CARTESIAN_POINT('Ctrl Pts',(7.09999865766138,1.31724253497577,0.641005923298765));
#16202=CARTESIAN_POINT('Ctrl Pts',(7.0999987494091,1.31399834762864,0.648240816253195));
#16203=CARTESIAN_POINT('Ctrl Pts',(7.09999933613984,1.30993159792479,0.655050690394837));
#16204=CARTESIAN_POINT('Ctrl Pts',(7.09999956222935,1.30510592187917,0.661272231165006));
#16205=CARTESIAN_POINT('Ctrl Pts',(7.09999960444598,1.30420484616769,0.662433950108221));
#16206=CARTESIAN_POINT('Ctrl Pts',(7.09999963060969,1.30327718139331,0.663575086117144));
#16207=CARTESIAN_POINT('Ctrl Pts',(7.09999963056866,1.30232317316131,0.664694459428815));
#16208=CARTESIAN_POINT('Ctrl Pts',(7.09999963048683,1.30042028596585,0.666927187690779));
#16209=CARTESIAN_POINT('Ctrl Pts',(7.09999952705857,1.29841262431024,0.669073382394206));
#16210=CARTESIAN_POINT('Ctrl Pts',(7.09999938633452,1.29630755303174,0.671129253595323));
#16211=CARTESIAN_POINT('Ctrl Pts',(7.09999900634735,1.29062337821964,0.676680576924663));
#16212=CARTESIAN_POINT('Ctrl Pts',(7.09999841760642,1.2842958957007,0.681513596217188));
#16213=CARTESIAN_POINT('Ctrl Pts',(7.0999982224057,1.2774887935492,0.68557385059291));
#16214=CARTESIAN_POINT('Ctrl Pts',(7.09999809840912,1.27316474526651,0.688153029745784));
#16215=CARTESIAN_POINT('Ctrl Pts',(7.09999810738417,1.26864620899217,0.690419707112974));
#16216=CARTESIAN_POINT('Ctrl Pts',(7.09999825155258,1.26396949224645,0.69235064530212));
#16217=CARTESIAN_POINT('Ctrl Pts',(7.09999847710269,1.25665281355793,0.695371579659609));
#16218=CARTESIAN_POINT('Ctrl Pts',(7.09999903441007,1.2490339950321,0.697538299034574));
#16219=CARTESIAN_POINT('Ctrl Pts',(7.09999948258254,1.24125996729125,0.698781081437474));
#16220=CARTESIAN_POINT('Ctrl Pts',(7.09999977198436,1.23623998534067,0.699583592753232));
#16221=CARTESIAN_POINT('Ctrl Pts',(7.1,1.23115469319345,0.7));
#16222=CARTESIAN_POINT('Ctrl Pts',(7.1,1.22604182196307,0.7));
#16223=CARTESIAN_POINT('Ctrl Pts',(7.1,1.35793097395724,0.));
#16224=CARTESIAN_POINT('Ctrl Pts',(7.1,1.35259441576718,0.100972845781549));
#16225=CARTESIAN_POINT('Ctrl Pts',(7.1,1.34725763161617,0.201946637598055));
#16226=CARTESIAN_POINT('Ctrl Pts',(7.1,1.33659371676552,0.403704849408333));
#16227=CARTESIAN_POINT('Ctrl Pts',(7.0999999994629,1.33126648576411,0.504491180117376));
#16228=CARTESIAN_POINT('Ctrl Pts',(7.0999999994629,1.32593912634735,0.605276549957215));
#16229=CARTESIAN_POINT('Ctrl Pts',(7.11011156210589,-1.35766432821499,-9.27062925672982E-5));
#16230=CARTESIAN_POINT('Ctrl Pts',(7.10674110347764,-1.34708925835705,0.201697046690488));
#16231=CARTESIAN_POINT('Ctrl Pts',(7.10337058314201,-1.33651419103807,0.403486798779133));
#16232=CARTESIAN_POINT('Ctrl Pts',(7.09999999999996,-1.32593912631822,0.605276549958221));
#16233=CARTESIAN_POINT('Ctrl Pts',(5.9694837631095,-1.38835096090528,2.80675674898241E-6));
#16234=CARTESIAN_POINT('Ctrl Pts',(5.96835662351021,-1.37777563343505,0.201792740207853));
#16235=CARTESIAN_POINT('Ctrl Pts',(5.96722945517891,-1.3672003004237,0.40358267322573));
#16236=CARTESIAN_POINT('Ctrl Pts',(5.96610224583462,-1.35662497356325,0.605372606931572));
#16237=CARTESIAN_POINT('Ctrl Pts',(4.8294200007394,-1.39866452387306,3.01102374082134E-5));
#16238=CARTESIAN_POINT('Ctrl Pts',(4.83053730380309,-1.38808904115766,0.201820093264151));
#16239=CARTESIAN_POINT('Ctrl Pts',(4.83165461298617,-1.3775135517806,0.403610075973038));
#16240=CARTESIAN_POINT('Ctrl Pts',(4.83277191472125,-1.36693806692183,0.605400059795761));
#16241=CARTESIAN_POINT('Ctrl Pts',(3.68991216363982,-1.37907703205181,-6.2684699445455E-5));
#16242=CARTESIAN_POINT('Ctrl Pts',(3.69327498756969,-1.36850179198701,0.201727122618256));
#16243=CARTESIAN_POINT('Ctrl Pts',(3.69663785098144,-1.3579265529724,0.403516929334346));
#16244=CARTESIAN_POINT('Ctrl Pts',(3.70000075457889,-1.34735131503281,0.605306735438421));
#16245=CARTESIAN_POINT('Ctrl Pts',(3.69999999992215,-1.34735368792773,0.6052614572053));
#16246=CARTESIAN_POINT('Ctrl Pts',(4.83355316856959,-1.366961322855,0.605214762857233));
#16247=CARTESIAN_POINT('Ctrl Pts',(5.96724522208681,-1.35660163688233,0.605228569880684));
#16248=CARTESIAN_POINT('Ctrl Pts',(7.09999999927392,-1.32593912632169,0.605276549957417));
#16249=CARTESIAN_POINT('Ctrl Pts',(7.1,-1.22604182196307,0.7));
#16250=CARTESIAN_POINT('Ctrl Pts',(5.96696284938742,-1.25674179781664,0.7));
#16251=CARTESIAN_POINT('Ctrl Pts',(4.83327074934872,-1.26710800714677,0.7));
#16252=CARTESIAN_POINT('Ctrl Pts',(3.7,-1.24747724070879,0.7));
#16253=CARTESIAN_POINT('Ctrl Pts',(7.10078315634008,-1.25494559805327,0.7));
#16254=CARTESIAN_POINT('Ctrl Pts',(5.96739926106349,-1.28566432005869,0.700000343763215));
#16255=CARTESIAN_POINT('Ctrl Pts',(4.83328164159484,-1.29603890521481,0.700000334703603));
#16256=CARTESIAN_POINT('Ctrl Pts',(3.69949916377151,-1.27639017438114,0.7));
#16257=CARTESIAN_POINT('Ctrl Pts',(7.10214055788579,-1.30504291366416,0.676629771601708));
#16258=CARTESIAN_POINT('Ctrl Pts',(5.96815960929481,-1.33579288254824,0.676614006760374));
#16259=CARTESIAN_POINT('Ctrl Pts',(4.83329467960724,-1.3461818279488,0.676609489640654));
#16260=CARTESIAN_POINT('Ctrl Pts',(3.69863109538965,-1.3265031696486,0.676624836591801));
#16261=CARTESIAN_POINT('Ctrl Pts',(7.10267376869946,-1.32472200604796,0.626932241521275));
#16262=CARTESIAN_POINT('Ctrl Pts',(5.9684558952243,-1.35546668061705,0.626891484245174));
#16263=CARTESIAN_POINT('Ctrl Pts',(4.83330292199863,-1.36585610284781,0.626879766983475));
#16264=CARTESIAN_POINT('Ctrl Pts',(3.69829020046733,-1.34618280086838,0.626919440930842));
#16265=CARTESIAN_POINT('Ctrl Pts',(7.10270476209941,-1.32586587253612,0.605276664588022));
#16266=CARTESIAN_POINT('Ctrl Pts',(5.96847377630401,-1.35660073810322,0.605228567467576));
#16267=CARTESIAN_POINT('Ctrl Pts',(4.8333022084086,-1.36698748587873,0.605214711607465));
#16268=CARTESIAN_POINT('Ctrl Pts',(3.69827043673666,-1.34732374755196,0.60526152849799));
#16269=CARTESIAN_POINT('Ctrl Pts',(7.1,-1.22604182196307,0.7));
#16270=CARTESIAN_POINT('Ctrl Pts',(5.96696284938742,-1.25674179781664,0.7));
#16271=CARTESIAN_POINT('Ctrl Pts',(4.83327074934872,-1.26710800714677,0.7));
#16272=CARTESIAN_POINT('Ctrl Pts',(3.7,-1.24747724070879,0.7));
#16273=CARTESIAN_POINT('Origin',(5.4,-8.11656130105013E-18,0.7));
#16274=CARTESIAN_POINT('Ctrl Pts',(3.7,1.24747724070879,0.7));
#16275=CARTESIAN_POINT('Ctrl Pts',(4.83327074934871,1.26710800714677,0.7));
#16276=CARTESIAN_POINT('Ctrl Pts',(5.96696284938742,1.25674179781664,0.7));
#16277=CARTESIAN_POINT('Ctrl Pts',(7.1,1.22604182196307,0.7));
#16278=CARTESIAN_POINT('Ctrl Pts',(3.7,1.24747724070879,0.7));
#16279=CARTESIAN_POINT('Ctrl Pts',(4.83327074934871,1.26710800714677,0.7));
#16280=CARTESIAN_POINT('Ctrl Pts',(5.96696284938742,1.25674179781664,0.7));
#16281=CARTESIAN_POINT('Ctrl Pts',(7.1,1.22604182196307,0.7));
#16282=CARTESIAN_POINT('Ctrl Pts',(3.69949916377151,1.27639017438114,0.7));
#16283=CARTESIAN_POINT('Ctrl Pts',(4.83328164159484,1.29603890521481,0.700000334703603));
#16284=CARTESIAN_POINT('Ctrl Pts',(5.96739926106349,1.28566432005869,0.700000343763215));
#16285=CARTESIAN_POINT('Ctrl Pts',(7.10078315634008,1.25494559805327,0.7));
#16286=CARTESIAN_POINT('Ctrl Pts',(3.69863109538965,1.3265031696486,0.676624836591801));
#16287=CARTESIAN_POINT('Ctrl Pts',(4.83329467960724,1.3461818279488,0.676609489640654));
#16288=CARTESIAN_POINT('Ctrl Pts',(5.9681596092948,1.33579288254824,0.676614006760374));
#16289=CARTESIAN_POINT('Ctrl Pts',(7.10214055788579,1.30504291366416,0.676629771601707));
#16290=CARTESIAN_POINT('Ctrl Pts',(3.69829020046733,1.34618280086838,0.626919440930842));
#16291=CARTESIAN_POINT('Ctrl Pts',(4.83330292199863,1.36585610284781,0.626879766983475));
#16292=CARTESIAN_POINT('Ctrl Pts',(5.9684558952243,1.35546668061705,0.626891484245174));
#16293=CARTESIAN_POINT('Ctrl Pts',(7.10267376869946,1.32472200604796,0.626932241521275));
#16294=CARTESIAN_POINT('Ctrl Pts',(3.69827043673666,1.34732374755196,0.60526152849799));
#16295=CARTESIAN_POINT('Ctrl Pts',(4.83330220840859,1.36698748587873,0.605214711607465));
#16296=CARTESIAN_POINT('Ctrl Pts',(5.96847377630401,1.35660073810322,0.605228567467576));
#16297=CARTESIAN_POINT('Ctrl Pts',(7.10270476209941,1.32586587253612,0.605276664588022));
#16298=CARTESIAN_POINT('Ctrl Pts',(7.09999999927392,1.32593912632169,0.605276549957417));
#16299=CARTESIAN_POINT('Ctrl Pts',(5.96724522208681,1.35660163688233,0.605228569880684));
#16300=CARTESIAN_POINT('Ctrl Pts',(4.83355316856959,1.366961322855,0.605214762857233));
#16301=CARTESIAN_POINT('Ctrl Pts',(3.69999999992215,1.34735368792773,0.6052614572053));
#16302=CARTESIAN_POINT('Ctrl Pts',(3.68991216360307,1.37907703216746,-6.26869063400631E-5));
#16303=CARTESIAN_POINT('Ctrl Pts',(3.6932749875452,1.36850179206412,0.201727121146993));
#16304=CARTESIAN_POINT('Ctrl Pts',(3.69663785096921,1.35792655301095,0.403516928598715));
#16305=CARTESIAN_POINT('Ctrl Pts',(3.70000075457892,1.34735131503281,0.605306735438421));
#16306=CARTESIAN_POINT('Ctrl Pts',(4.8294200007272,1.39866452398872,3.01080305115927E-5));
#16307=CARTESIAN_POINT('Ctrl Pts',(4.83053730379496,1.38808904123477,0.201820091792887));
#16308=CARTESIAN_POINT('Ctrl Pts',(4.83165461298211,1.37751355181915,0.403610075237406));
#16309=CARTESIAN_POINT('Ctrl Pts',(4.83277191472127,1.36693806692183,0.605400059795761));
#16310=CARTESIAN_POINT('Ctrl Pts',(5.96948376312183,1.38835096102094,2.80454985295556E-6));
#16311=CARTESIAN_POINT('Ctrl Pts',(5.96835662351844,1.37777563351215,0.201792738736588));
#16312=CARTESIAN_POINT('Ctrl Pts',(5.96722945518303,1.36720030046225,0.403582672490098));
#16313=CARTESIAN_POINT('Ctrl Pts',(5.96610224583462,1.35662497356325,0.605372606931572));
#16314=CARTESIAN_POINT('Ctrl Pts',(7.11011156214274,1.35766432833065,-9.27084994613511E-5));
#16315=CARTESIAN_POINT('Ctrl Pts',(7.10674110350221,1.34708925843416,0.201697045219225));
#16316=CARTESIAN_POINT('Ctrl Pts',(7.10337058315429,1.33651419107662,0.403486798043502));
#16317=CARTESIAN_POINT('Ctrl Pts',(7.09999999999996,1.32593912631822,0.605276549958221));
#16318=CARTESIAN_POINT('Origin',(3.5,1.44777777777778,0.));
#16319=CARTESIAN_POINT('',(3.5,-1.34358136363184,0.605270327458634));
#16320=CARTESIAN_POINT('Ctrl Pts',(3.5,-1.34358136363184,0.605270327458634));
#16321=CARTESIAN_POINT('Ctrl Pts',(3.5,-1.34890136370362,0.504489156176152));
#16322=CARTESIAN_POINT('Ctrl Pts',(3.5,-1.35422123464986,0.403706701640381));
#16323=CARTESIAN_POINT('Ctrl Pts',(3.5,-1.3648706701715,0.201950780690867));
#16324=CARTESIAN_POINT('Ctrl Pts',(3.5,-1.3702003690246,0.100974756199658));
#16325=CARTESIAN_POINT('Ctrl Pts',(3.5,-1.37552980833516,0.));
#16326=CARTESIAN_POINT('',(3.5,-1.24369946473884,0.7));
#16327=CARTESIAN_POINT('Ctrl Pts',(3.49999999991873,-1.24369946470729,0.7));
#16328=CARTESIAN_POINT('Ctrl Pts',(3.49999999896975,-1.25160831520001,0.699999999810925));
#16329=CARTESIAN_POINT('Ctrl Pts',(3.50000040534574,-1.25945374057332,0.69900619751828));
#16330=CARTESIAN_POINT('Ctrl Pts',(3.50000075715473,-1.26709539726361,0.697119355224275));
#16331=CARTESIAN_POINT('Ctrl Pts',(3.5000009551612,-1.27139630362835,0.696057395447694));
#16332=CARTESIAN_POINT('Ctrl Pts',(3.50000113454144,-1.27563271975905,0.694711510656402));
#16333=CARTESIAN_POINT('Ctrl Pts',(3.50000124621709,-1.27977793997275,0.693092697679401));
#16334=CARTESIAN_POINT('Ctrl Pts',(3.50000144618968,-1.28720060051191,0.690193961644836));
#16335=CARTESIAN_POINT('Ctrl Pts',(3.50000138985083,-1.29425038514255,0.686454755369034));
#16336=CARTESIAN_POINT('Ctrl Pts',(3.5000011147959,-1.30078112659466,0.681956784255818));
#16337=CARTESIAN_POINT('Ctrl Pts',(3.50000096334461,-1.30437709646577,0.679480102439082));
#16338=CARTESIAN_POINT('Ctrl Pts',(3.50000075087427,-1.30781543681835,0.676772489296601));
#16339=CARTESIAN_POINT('Ctrl Pts',(3.50000056308077,-1.31106783354026,0.67384203444854));
#16340=CARTESIAN_POINT('Ctrl Pts',(3.50000037990614,-1.31424023611357,0.670983655445047));
#16341=CARTESIAN_POINT('Ctrl Pts',(3.50000021841608,-1.31721646102264,0.667930553458483));
#16342=CARTESIAN_POINT('Ctrl Pts',(3.50000022028926,-1.3199739184757,0.664694242102541));
#16343=CARTESIAN_POINT('Ctrl Pts',(3.50000022375892,-1.32508151834405,0.658699667848218));
#16344=CARTESIAN_POINT('Ctrl Pts',(3.50000072745304,-1.32944146850927,0.652077914129702));
#16345=CARTESIAN_POINT('Ctrl Pts',(3.50000090782832,-1.33299465793893,0.64499486611401));
#16346=CARTESIAN_POINT('Ctrl Pts',(3.50000092626355,-1.33335781125732,0.644270944003422));
#16347=CARTESIAN_POINT('Ctrl Pts',(3.50000094214549,-1.33371249714824,0.643542183465449));
#16348=CARTESIAN_POINT('Ctrl Pts',(3.5000009551778,-1.33405862411533,0.642808750463418));
#16349=CARTESIAN_POINT('Ctrl Pts',(3.50000108270827,-1.3374457225345,0.635631587173848));
#16350=CARTESIAN_POINT('Ctrl Pts',(3.5000008470667,-1.33997810357527,0.628091493562486));
#16351=CARTESIAN_POINT('Ctrl Pts',(3.50000049017339,-1.34160279315579,0.620357239364781));
#16352=CARTESIAN_POINT('Ctrl Pts',(3.50000026118253,-1.3426452308862,0.615394766232079));
#16353=CARTESIAN_POINT('Ctrl Pts',(3.5,-1.34331313055125,0.610351689051435));
#16354=CARTESIAN_POINT('Ctrl Pts',(3.5,-1.34358136363184,0.605270327458634));
#16355=CARTESIAN_POINT('',(3.5,0.723888888888889,0.7));
#16356=CARTESIAN_POINT('Ctrl Pts',(3.5,1.37552980833516,0.));
#16357=CARTESIAN_POINT('Ctrl Pts',(3.5,1.37020035376703,0.10097504527886));
#16358=CARTESIAN_POINT('Ctrl Pts',(3.5,1.36487063968137,0.201951358354439));
#16359=CARTESIAN_POINT('Ctrl Pts',(3.5,1.35422120417274,0.403707279015233));
#16360=CARTESIAN_POINT('Ctrl Pts',(3.5,1.34890134846466,0.504489444860456));
#16361=CARTESIAN_POINT('Ctrl Pts',(3.5,1.34358136363184,0.605270327458635));
#16362=CARTESIAN_POINT('Ctrl Pts',(3.50000000097418,-1.37552980835478,3.46944695195361E-18));
#16363=CARTESIAN_POINT('Ctrl Pts',(3.50374047168104,-1.36494504174376,0.201972406882836));
#16364=CARTESIAN_POINT('Ctrl Pts',(3.50748098869546,-1.35436027657305,0.403944812985359));
#16365=CARTESIAN_POINT('Ctrl Pts',(3.51122155284351,-1.34377551287676,0.605917218294091));
#16366=CARTESIAN_POINT('Ctrl Pts',(2.69119625874569,-1.35924722858667,-7.54309614812119E-5));
#16367=CARTESIAN_POINT('Ctrl Pts',(2.69653217397324,-1.34866266892899,0.20189683354744));
#16368=CARTESIAN_POINT('Ctrl Pts',(2.70186816749714,-1.3380781117335,0.403869096002786));
#16369=CARTESIAN_POINT('Ctrl Pts',(2.7072042346663,-1.32749355863083,0.605841357314298));
#16370=CARTESIAN_POINT('Ctrl Pts',(1.88267190563219,-1.32763345268679,-0.000212792412547521));
#16371=CARTESIAN_POINT('Ctrl Pts',(1.88960380459144,-1.31704931403188,0.201759213581099));
#16372=CARTESIAN_POINT('Ctrl Pts',(1.89653581411498,-1.30646518166523,0.403731216009517));
#16373=CARTESIAN_POINT('Ctrl Pts',(1.90346792975642,-1.29588105699583,0.605703215867581));
#16374=CARTESIAN_POINT('Ctrl Pts',(1.07441451989529,-1.27728918272486,-0.000429194541766893));
#16375=CARTESIAN_POINT('Ctrl Pts',(1.08294287068452,-1.26670581246828,0.201542410257184));
#16376=CARTESIAN_POINT('Ctrl Pts',(1.09147136321593,-1.25612245578053,0.403514009799157));
#16377=CARTESIAN_POINT('Ctrl Pts',(1.09999999999989,-1.24553911298205,0.605485603995245));
#16378=CARTESIAN_POINT('Ctrl Pts',(1.09999999916631,-1.24553911263844,0.605485603997431));
#16379=CARTESIAN_POINT('Ctrl Pts',(1.89930203168262,-1.29563783986497,0.605377360150118));
#16380=CARTESIAN_POINT('Ctrl Pts',(2.69958486793449,-1.32722445934619,0.605308375488923));
#16381=CARTESIAN_POINT('Ctrl Pts',(3.5,-1.34358136363184,0.605270327458634));
#16382=CARTESIAN_POINT('Ctrl Pts',(3.50204003610941,-1.24374118183538,0.7));
#16383=CARTESIAN_POINT('Ctrl Pts',(2.70080437300401,-1.2273695200909,0.7));
#16384=CARTESIAN_POINT('Ctrl Pts',(1.89984199608574,-1.1957170361627,0.7));
#16385=CARTESIAN_POINT('Ctrl Pts',(1.1,-1.14549341399196,0.7));
#16386=CARTESIAN_POINT('Ctrl Pts',(3.50144932661635,-1.27265074030048,0.7));
#16387=CARTESIAN_POINT('Ctrl Pts',(2.6998452019678,-1.25626413437997,0.699999727319846));
#16388=CARTESIAN_POINT('Ctrl Pts',(1.89847848223078,-1.22458382597074,0.70000077422621));
#16389=CARTESIAN_POINT('Ctrl Pts',(1.09819048660397,-1.17431102498992,0.7));
#16390=CARTESIAN_POINT('Ctrl Pts',(3.50042536655637,-1.322763754511,0.676632802377821));
#16391=CARTESIAN_POINT('Ctrl Pts',(2.69818680938114,-1.3063522351595,0.67664530655333));
#16392=CARTESIAN_POINT('Ctrl Pts',(1.89610976425884,-1.27462253270773,0.67666760713801));
#16393=CARTESIAN_POINT('Ctrl Pts',(1.09505363188407,-1.22426736091617,0.676703190608825));
#16394=CARTESIAN_POINT('Ctrl Pts',(3.50002334924346,-1.34243864233338,0.626926882269943));
#16395=CARTESIAN_POINT('Ctrl Pts',(2.6975332861013,-1.32603127467068,0.626959208652505));
#16396=CARTESIAN_POINT('Ctrl Pts',(1.89518106151152,-1.29430885982199,0.62701751976321));
#16397=CARTESIAN_POINT('Ctrl Pts',(1.09381704710221,-1.24396073223232,0.627109609335854));
#16398=CARTESIAN_POINT('Ctrl Pts',(3.5,-1.34358136363184,0.605270327458634));
#16399=CARTESIAN_POINT('Ctrl Pts',(2.69749615303,-1.32718177535833,0.605308474776761));
#16400=CARTESIAN_POINT('Ctrl Pts',(1.89512529323683,-1.29547288309274,0.605377720397184));
#16401=CARTESIAN_POINT('Ctrl Pts',(1.09374258853658,-1.24514653057163,0.605486452199395));
#16402=CARTESIAN_POINT('Ctrl Pts',(3.49999999991875,-1.24369946470729,0.7));
#16403=CARTESIAN_POINT('Ctrl Pts',(3.26917843083003,-1.23897560807887,0.7));
#16404=CARTESIAN_POINT('Ctrl Pts',(3.03837960179139,-1.23298334389983,0.7));
#16405=CARTESIAN_POINT('Ctrl Pts',(2.80762376541487,-1.22564400623233,0.7));
#16406=CARTESIAN_POINT('Ctrl Pts',(2.57739190516312,-1.2178709162388,0.7));
#16407=CARTESIAN_POINT('Ctrl Pts',(2.08463535466707,-1.20026407570248,0.7));
#16408=CARTESIAN_POINT('Ctrl Pts',(1.59210562457525,-1.17639367564078,0.7));
#16409=CARTESIAN_POINT('Ctrl Pts',(1.1,-1.14549341399196,0.7));
#16410=CARTESIAN_POINT('Origin',(5.4,-8.11656130105013E-18,0.7));
#16411=CARTESIAN_POINT('Ctrl Pts',(1.0744145198953,1.27728918272486,-0.000429194541767127));
#16412=CARTESIAN_POINT('Ctrl Pts',(1.08294287068452,1.26670581246828,0.201542410257184));
#16413=CARTESIAN_POINT('Ctrl Pts',(1.09147136321593,1.25612245578053,0.403514009799157));
#16414=CARTESIAN_POINT('Ctrl Pts',(1.0999999999999,1.24553911298205,0.605485603995245));
#16415=CARTESIAN_POINT('Ctrl Pts',(1.88267190563235,1.3276334526868,-0.000212792412547728));
#16416=CARTESIAN_POINT('Ctrl Pts',(1.8896038045916,1.31704931403189,0.201759213581098));
#16417=CARTESIAN_POINT('Ctrl Pts',(1.89653581411514,1.30646518166524,0.403731216009517));
#16418=CARTESIAN_POINT('Ctrl Pts',(1.90346792975658,1.29588105699584,0.605703215867581));
#16419=CARTESIAN_POINT('Ctrl Pts',(2.69119625874601,1.35924722858668,-7.54309614812134E-5));
#16420=CARTESIAN_POINT('Ctrl Pts',(2.69653217397356,1.348662668929,0.201896833547441));
#16421=CARTESIAN_POINT('Ctrl Pts',(2.70186816749745,1.33807811173351,0.403869096002786));
#16422=CARTESIAN_POINT('Ctrl Pts',(2.70720423466661,1.32749355863085,0.605841357314298));
#16423=CARTESIAN_POINT('Ctrl Pts',(3.50000000097466,1.37552980835479,-3.81639164714898E-17));
#16424=CARTESIAN_POINT('Ctrl Pts',(3.50374047168151,1.36494504174377,0.201972406882836));
#16425=CARTESIAN_POINT('Ctrl Pts',(3.50748098869594,1.35436027657306,0.403944812985359));
#16426=CARTESIAN_POINT('Ctrl Pts',(3.51122155284398,1.34377551287677,0.605917218294091));
#16427=CARTESIAN_POINT('Origin',(0.9,1.34328341716202,0.));
#16428=CARTESIAN_POINT('',(0.9,-1.23261418131727,0.605513513251856));
#16429=CARTESIAN_POINT('Ctrl Pts',(0.9,-1.23261418131727,0.605513513251856));
#16430=CARTESIAN_POINT('Ctrl Pts',(0.9,-1.23820195798151,0.504544236118289));
#16431=CARTESIAN_POINT('Ctrl Pts',(0.9,-1.24378834611607,0.403573587101897));
#16432=CARTESIAN_POINT('Ctrl Pts',(0.9,-1.25495246062481,0.201736610752668));
#16433=CARTESIAN_POINT('Ctrl Pts',(0.9,-1.26053033259331,0.100867703930409));
#16434=CARTESIAN_POINT('Ctrl Pts',(0.9,-1.266106713614,0.));
#16435=CARTESIAN_POINT('',(0.9,-1.13254484134404,0.7));
#16436=CARTESIAN_POINT('Ctrl Pts',(0.899999999937205,-1.13254484130906,
0.7));
#16437=CARTESIAN_POINT('Ctrl Pts',(0.899999996287105,-1.14047016437301,
0.699999998205918));
#16438=CARTESIAN_POINT('Ctrl Pts',(0.900001280561548,-1.14833327216777,
0.699006663725481));
#16439=CARTESIAN_POINT('Ctrl Pts',(0.900002371513522,-1.15599299513142,
0.697119896446058));
#16440=CARTESIAN_POINT('Ctrl Pts',(0.900002982478546,-1.16028266409831,
0.696063251566776));
#16441=CARTESIAN_POINT('Ctrl Pts',(0.900003528700818,-1.16450859688491,
0.694725368779139));
#16442=CARTESIAN_POINT('Ctrl Pts',(0.900003857331964,-1.16864431737637,
0.693116947675672));
#16443=CARTESIAN_POINT('Ctrl Pts',(0.900004447924614,-1.17607674172948,
0.690226407030055));
#16444=CARTESIAN_POINT('Ctrl Pts',(0.900004211500339,-1.18313828052408,
0.686496282267003));
#16445=CARTESIAN_POINT('Ctrl Pts',(0.900003280035406,-1.18968205680082,
0.682006679400108));
#16446=CARTESIAN_POINT('Ctrl Pts',(0.900002768383153,-1.19327654302499,
0.679540547464272));
#16447=CARTESIAN_POINT('Ctrl Pts',(0.900002064672634,-1.19671453445753,
0.676844382327844));
#16448=CARTESIAN_POINT('Ctrl Pts',(0.900001450170085,-1.19996775918788,
0.673925988054463));
#16449=CARTESIAN_POINT('Ctrl Pts',(0.900000850201302,-1.20314404102283,
0.67107661751105));
#16450=CARTESIAN_POINT('Ctrl Pts',(0.900000329673364,-1.20612495630093,
0.668032594545539));
#16451=CARTESIAN_POINT('Ctrl Pts',(0.900000346081477,-1.20888784276431,
0.664805176146368));
#16452=CARTESIAN_POINT('Ctrl Pts',(0.900000376514472,-1.21401231436848,
0.658819112599938));
#16453=CARTESIAN_POINT('Ctrl Pts',(0.900002057232535,-1.21838968018573,
0.652203523053766));
#16454=CARTESIAN_POINT('Ctrl Pts',(0.900002698394847,-1.22195969054856,
0.645123732731769));
#16455=CARTESIAN_POINT('Ctrl Pts',(0.900002763240662,-1.22232075393107,
0.644407697543824));
#16456=CARTESIAN_POINT('Ctrl Pts',(0.90000282009371,-1.22267351953901,0.643686895083047));
#16457=CARTESIAN_POINT('Ctrl Pts',(0.900002868017411,-1.22301789747605,
0.642961485862499));
#16458=CARTESIAN_POINT('Ctrl Pts',(0.900003341628975,-1.22642125256928,
0.635792544708285));
#16459=CARTESIAN_POINT('Ctrl Pts',(0.900002645022176,-1.22896979279554,
0.628258742918086));
#16460=CARTESIAN_POINT('Ctrl Pts',(0.900001532827652,-1.23061007098772,
0.6205286650049));
#16461=CARTESIAN_POINT('Ctrl Pts',(0.900000822323555,-1.23165793118585,
0.61559045329652));
#16462=CARTESIAN_POINT('Ctrl Pts',(0.900000000000001,-1.23233426661673,
0.610571479357261));
#16463=CARTESIAN_POINT('Ctrl Pts',(0.900000000000001,-1.23261418131727,
0.605513513251856));
#16464=CARTESIAN_POINT('',(0.9,1.13254484134404,0.7));
#16465=CARTESIAN_POINT('',(0.9,0.671641708581009,0.7));
#16466=CARTESIAN_POINT('',(0.9,1.23261418131727,0.605513513251856));
#16467=CARTESIAN_POINT('Ctrl Pts',(0.9,1.23261418131727,0.605513513251856));
#16468=CARTESIAN_POINT('Ctrl Pts',(0.9,1.23217633603244,0.613425232807268));
#16469=CARTESIAN_POINT('Ctrl Pts',(0.900001832787994,1.23077105609892,0.621244170085157));
#16470=CARTESIAN_POINT('Ctrl Pts',(0.900002580745575,1.22848219166492,0.628809599741497));
#16471=CARTESIAN_POINT('Ctrl Pts',(0.900002993068559,1.22722042035689,0.632980157827643));
#16472=CARTESIAN_POINT('Ctrl Pts',(0.90000314174678,1.22568915198244,0.637073706995481));
#16473=CARTESIAN_POINT('Ctrl Pts',(0.900002971484041,1.2238959908032,0.641061424759933));
#16474=CARTESIAN_POINT('Ctrl Pts',(0.900002662567364,1.22064256379503,0.648296551655426));
#16475=CARTESIAN_POINT('Ctrl Pts',(0.900001146653719,1.21656554418039,0.655104870690721));
#16476=CARTESIAN_POINT('Ctrl Pts',(0.900000540233788,1.21172928299109,0.66132323772617));
#16477=CARTESIAN_POINT('Ctrl Pts',(0.900000424918953,1.21080963534652,0.66250570210793));
#16478=CARTESIAN_POINT('Ctrl Pts',(0.900000351402035,1.20986240082127,0.663666762843393));
#16479=CARTESIAN_POINT('Ctrl Pts',(0.900000346234225,1.20888784277449,0.664805176146358));
#16480=CARTESIAN_POINT('Ctrl Pts',(0.900000336405833,1.20703438079614,0.666970266034709));
#16481=CARTESIAN_POINT('Ctrl Pts',(0.900000571869483,1.20508211779724,0.669053482241208));
#16482=CARTESIAN_POINT('Ctrl Pts',(0.900000903580486,1.20303784749416,0.671051418948595));
#16483=CARTESIAN_POINT('Ctrl Pts',(0.900001825932764,1.19735357006848,0.676606861644505));
#16484=CARTESIAN_POINT('Ctrl Pts',(0.900003332967427,1.19102482074992,0.681443262092019));
#16485=CARTESIAN_POINT('Ctrl Pts',(0.900003895332687,1.18421635668109,0.685507797106414));
#16486=CARTESIAN_POINT('Ctrl Pts',(0.900004254598985,1.17986677848026,0.688104419886002));
#16487=CARTESIAN_POINT('Ctrl Pts',(0.9000042929279,1.17532044218795,0.69038534615497));
#16488=CARTESIAN_POINT('Ctrl Pts',(0.900003997675654,1.17061445353731,0.692327416690341));
#16489=CARTESIAN_POINT('Ctrl Pts',(0.900003537640084,1.16328200409216,0.695353376818313));
#16490=CARTESIAN_POINT('Ctrl Pts',(0.900002259964378,1.15564663185935,0.697524398440697));
#16491=CARTESIAN_POINT('Ctrl Pts',(0.900001215101098,1.14785635641255,0.698771715080855));
#16492=CARTESIAN_POINT('Ctrl Pts',(0.900000537649455,1.14280542295857,0.699580430175527));
#16493=CARTESIAN_POINT('Ctrl Pts',(0.899999997568109,1.13768876957788,0.699999998835552));
#16494=CARTESIAN_POINT('Ctrl Pts',(0.899999999937205,1.13254484130906,0.7));
#16495=CARTESIAN_POINT('Ctrl Pts',(0.9,1.266106713614,0.));
#16496=CARTESIAN_POINT('Ctrl Pts',(0.9,1.26053025554556,0.100869097599589));
#16497=CARTESIAN_POINT('Ctrl Pts',(0.9,1.25495230648558,0.201739398169819));
#16498=CARTESIAN_POINT('Ctrl Pts',(0.9,1.24378819189631,0.403576374532447));
#16499=CARTESIAN_POINT('Ctrl Pts',(0.9,1.23820188085298,0.504545629805417));
#16500=CARTESIAN_POINT('Ctrl Pts',(0.9,1.23261418131727,0.605513513251856));
#16501=CARTESIAN_POINT('Ctrl Pts',(0.900000000000002,-1.266106713614,-8.15320033709099E-17));
#16502=CARTESIAN_POINT('Ctrl Pts',(0.908871090277923,-1.25552568177643,
0.201930159665972));
#16503=CARTESIAN_POINT('Ctrl Pts',(0.917742329685194,-1.24494466498547,
0.403860313587921));
#16504=CARTESIAN_POINT('Ctrl Pts',(0.926613720860141,-1.23436366359623,
0.605790461668883));
#16505=CARTESIAN_POINT('Ctrl Pts',(0.697441255022372,-1.25280938151844,
-5.71013218131409E-5));
#16506=CARTESIAN_POINT('Ctrl Pts',(0.706712389899261,-1.24222855501813,
0.201872952723963));
#16507=CARTESIAN_POINT('Ctrl Pts',(0.71598368260269,-1.23164774534186,0.403803000441224));
#16508=CARTESIAN_POINT('Ctrl Pts',(0.725255135891715,-1.22106695288555,
0.605733041729342));
#16509=CARTESIAN_POINT('Ctrl Pts',(0.494899146035781,-1.23832021354117,
-0.000119230777047918));
#16510=CARTESIAN_POINT('Ctrl Pts',(0.504570354086872,-1.2277396148863,0.201810708652083));
#16511=CARTESIAN_POINT('Ctrl Pts',(0.514241728780064,-1.21715903502506,
0.403740641123913));
#16512=CARTESIAN_POINT('Ctrl Pts',(0.523913273026478,-1.20657847439907,
0.605670566527588));
#16513=CARTESIAN_POINT('Ctrl Pts',(0.292373353339556,-1.22258574808743,
-0.000186633859775947));
#16514=CARTESIAN_POINT('Ctrl Pts',(0.302444661323169,-1.21200540195431,
0.201743181663441));
#16515=CARTESIAN_POINT('Ctrl Pts',(0.312516144861689,-1.20142507679253,
0.403672989556125));
#16516=CARTESIAN_POINT('Ctrl Pts',(0.322587807049886,-1.190844773096,0.605602789690272));
#16517=CARTESIAN_POINT('',(0.32407846024449,-1.19096124572524,0.605603291426262));
#16518=CARTESIAN_POINT('Ctrl Pts',(0.292382661757373,-1.22257596919059,
-1.26634813746307E-16));
#16519=CARTESIAN_POINT('Ctrl Pts',(0.302948004341657,-1.21203750712027,
0.201867748891544));
#16520=CARTESIAN_POINT('Ctrl Pts',(0.313513270922098,-1.20149926476964,
0.403735512620674));
#16521=CARTESIAN_POINT('Ctrl Pts',(0.324078460244491,-1.19096124572524,
0.605603291426262));
#16522=CARTESIAN_POINT('Ctrl Pts',(0.324078460244487,-1.19096124572524,
0.605603291426262));
#16523=CARTESIAN_POINT('Ctrl Pts',(0.515976798438381,-1.20595780001216,
0.605571001180369));
#16524=CARTESIAN_POINT('Ctrl Pts',(0.707956283694857,-1.21982772882273,
0.605541108414459));
#16525=CARTESIAN_POINT('Ctrl Pts',(0.900000000000001,-1.23261418131727,
0.605513513251856));
#16526=CARTESIAN_POINT('Ctrl Pts',(0.906632491847682,-1.13298681949577,
0.7));
#16527=CARTESIAN_POINT('Ctrl Pts',(0.714963137593258,-1.12022681655782,
0.7));
#16528=CARTESIAN_POINT('Ctrl Pts',(0.52336552158394,-1.10638609587519,0.7));
#16529=CARTESIAN_POINT('Ctrl Pts',(0.331856371369197,-1.09142177001972,
0.7));
#16530=CARTESIAN_POINT('Ctrl Pts',(0.904714827274509,-1.16179226195561,
0.7));
#16531=CARTESIAN_POINT('Ctrl Pts',(0.712937153454425,-1.14901967286075,
0.69999980360337));
#16532=CARTESIAN_POINT('Ctrl Pts',(0.521230340369869,-1.13516557394852,
0.700000229443053));
#16533=CARTESIAN_POINT('Ctrl Pts',(0.329608751265076,-1.12018616744754,
0.7));
#16534=CARTESIAN_POINT('Ctrl Pts',(0.901389714107723,-1.21173913866089,
0.676722045797292));
#16535=CARTESIAN_POINT('Ctrl Pts',(0.709425477581998,-1.19894546296063,
0.676731074746188));
#16536=CARTESIAN_POINT('Ctrl Pts',(0.517526696841433,-1.18506766126723,
0.67674067107047));
#16537=CARTESIAN_POINT('Ctrl Pts',(0.325711429829026,-1.17006296935233,
0.676751229163451));
#16538=CARTESIAN_POINT('Ctrl Pts',(0.900079298017777,-1.23142303740181,
0.627132481749528));
#16539=CARTESIAN_POINT('Ctrl Pts',(0.708040181852795,-1.21863106773591,
0.627155851652593));
#16540=CARTESIAN_POINT('Ctrl Pts',(0.516066269599777,-1.20475540724405,
0.627181012790208));
#16541=CARTESIAN_POINT('Ctrl Pts',(0.324172915772929,-1.18975243096407,
0.627208352638976));
#16542=CARTESIAN_POINT('Ctrl Pts',(0.900000000000001,-1.23261418131727,
0.605513513251856));
#16543=CARTESIAN_POINT('Ctrl Pts',(0.707956283694857,-1.21982772882273,
0.605541108414459));
#16544=CARTESIAN_POINT('Ctrl Pts',(0.515976798438381,-1.20595780001216,
0.605571001180369));
#16545=CARTESIAN_POINT('Ctrl Pts',(0.324078460244487,-1.19096124572524,
0.605603291426262));
#16546=CARTESIAN_POINT('',(0.3318563713692,-1.09142177001972,0.7));
#16547=CARTESIAN_POINT('Origin',(0.3318563713692,-1.09142177001972,0.6));
#16548=CARTESIAN_POINT('Ctrl Pts',(0.899999999937167,-1.13254484130906,
0.7));
#16549=CARTESIAN_POINT('Ctrl Pts',(0.710543123935439,-1.11990737114256,
0.7));
#16550=CARTESIAN_POINT('Ctrl Pts',(0.521156529292483,-1.10621348751457,
0.7));
#16551=CARTESIAN_POINT('Ctrl Pts',(0.331856371369197,-1.09142177001972,
0.7));
#16552=CARTESIAN_POINT('Origin',(5.4,-8.11656130105013E-18,0.7));
#16553=CARTESIAN_POINT('',(0.3318563713692,1.09142177001972,0.7));
#16554=CARTESIAN_POINT('',(0.3318563713692,-0.7,0.7));
#16555=CARTESIAN_POINT('Ctrl Pts',(0.3318563713692,1.09142177001972,0.7));
#16556=CARTESIAN_POINT('Ctrl Pts',(0.521156529292483,1.10621348751457,0.7));
#16557=CARTESIAN_POINT('Ctrl Pts',(0.710543123935438,1.11990737114256,0.7));
#16558=CARTESIAN_POINT('Ctrl Pts',(0.899999999937165,1.13254484130906,0.7));
#16559=CARTESIAN_POINT('Ctrl Pts',(0.292373353339556,1.22258574808743,-0.000186633859776018));
#16560=CARTESIAN_POINT('Ctrl Pts',(0.30244466132317,1.21200540195431,0.20174318166344));
#16561=CARTESIAN_POINT('Ctrl Pts',(0.31251614486169,1.20142507679253,0.403672989556124));
#16562=CARTESIAN_POINT('Ctrl Pts',(0.322587807049886,1.190844773096,0.605602789690271));
#16563=CARTESIAN_POINT('Ctrl Pts',(0.494899146035781,1.23832021354117,-0.000119230777047989));
#16564=CARTESIAN_POINT('Ctrl Pts',(0.504570354086872,1.2277396148863,0.201810708652083));
#16565=CARTESIAN_POINT('Ctrl Pts',(0.514241728780064,1.21715903502506,0.403740641123914));
#16566=CARTESIAN_POINT('Ctrl Pts',(0.523913273026478,1.20657847439907,0.605670566527587));
#16567=CARTESIAN_POINT('Ctrl Pts',(0.697441255022371,1.25280938151844,-5.71013218130602E-5));
#16568=CARTESIAN_POINT('Ctrl Pts',(0.70671238989926,1.24222855501813,0.201872952723963));
#16569=CARTESIAN_POINT('Ctrl Pts',(0.715983682602689,1.23164774534186,0.403803000441224));
#16570=CARTESIAN_POINT('Ctrl Pts',(0.725255135891714,1.22106695288555,0.605733041729342));
#16571=CARTESIAN_POINT('Ctrl Pts',(0.9,1.266106713614,1.73472347597681E-18));
#16572=CARTESIAN_POINT('Ctrl Pts',(0.908871090277921,1.25552568177643,0.201930159665973));
#16573=CARTESIAN_POINT('Ctrl Pts',(0.917742329685192,1.24494466498547,0.403860313587921));
#16574=CARTESIAN_POINT('Ctrl Pts',(0.92661372086014,1.23436366359623,0.605790461668883));
#16575=CARTESIAN_POINT('',(0.32407846024449,1.19096124572524,0.605603291426262));
#16576=CARTESIAN_POINT('Ctrl Pts',(0.9,1.23261418131727,0.605513513251856));
#16577=CARTESIAN_POINT('Ctrl Pts',(0.707956283694857,1.21982772882273,0.605541108414459));
#16578=CARTESIAN_POINT('Ctrl Pts',(0.515976798438382,1.20595780001216,0.60557100118037));
#16579=CARTESIAN_POINT('Ctrl Pts',(0.32407846024449,1.19096124572524,0.605603291426262));
#16580=CARTESIAN_POINT('Ctrl Pts',(0.324078460244491,1.19096124572524,0.605603291426262));
#16581=CARTESIAN_POINT('Ctrl Pts',(0.313513270922098,1.20149926476964,0.403735512620674));
#16582=CARTESIAN_POINT('Ctrl Pts',(0.302948004341658,1.21203750712026,0.201867748891544));
#16583=CARTESIAN_POINT('Ctrl Pts',(0.292382661757373,1.22257596919059,3.4477629085039E-17));
#16584=CARTESIAN_POINT('Ctrl Pts',(0.3318563713692,1.09142177001972,0.7));
#16585=CARTESIAN_POINT('Ctrl Pts',(0.523365521583941,1.10638609587519,0.7));
#16586=CARTESIAN_POINT('Ctrl Pts',(0.714963137593258,1.12022681655782,0.7));
#16587=CARTESIAN_POINT('Ctrl Pts',(0.906632491847681,1.13298681949577,0.7));
#16588=CARTESIAN_POINT('Ctrl Pts',(0.329608751265078,1.12018616744754,0.7));
#16589=CARTESIAN_POINT('Ctrl Pts',(0.52123034036987,1.13516557394852,0.700000229443053));
#16590=CARTESIAN_POINT('Ctrl Pts',(0.712937153454426,1.14901967286075,0.699999803603371));
#16591=CARTESIAN_POINT('Ctrl Pts',(0.904714827274509,1.16179226195561,0.700000000000001));
#16592=CARTESIAN_POINT('Ctrl Pts',(0.325711429829028,1.17006296935233,0.676751229163452));
#16593=CARTESIAN_POINT('Ctrl Pts',(0.517526696841433,1.18506766126723,0.67674067107047));
#16594=CARTESIAN_POINT('Ctrl Pts',(0.709425477581997,1.19894546296063,0.676731074746189));
#16595=CARTESIAN_POINT('Ctrl Pts',(0.901389714107722,1.21173913866089,0.676722045797292));
#16596=CARTESIAN_POINT('Ctrl Pts',(0.324172915772932,1.18975243096407,0.627208352638976));
#16597=CARTESIAN_POINT('Ctrl Pts',(0.516066269599778,1.20475540724405,0.627181012790208));
#16598=CARTESIAN_POINT('Ctrl Pts',(0.708040181852794,1.21863106773591,0.627155851652593));
#16599=CARTESIAN_POINT('Ctrl Pts',(0.900079298017776,1.23142303740181,0.627132481749528));
#16600=CARTESIAN_POINT('Ctrl Pts',(0.32407846024449,1.19096124572524,0.605603291426262));
#16601=CARTESIAN_POINT('Ctrl Pts',(0.515976798438382,1.20595780001216,0.60557100118037));
#16602=CARTESIAN_POINT('Ctrl Pts',(0.707956283694857,1.21982772882273,0.605541108414459));
#16603=CARTESIAN_POINT('Ctrl Pts',(0.9,1.23261418131727,0.605513513251856));
#16604=CARTESIAN_POINT('Origin',(0.331856371369202,1.09142177001972,0.6));
#16605=CARTESIAN_POINT('Origin',(0.331856371369202,1.09142177001972,0.6));
#16606=CARTESIAN_POINT('Origin',(0.331856371369201,1.09142177001972,0.6));
#16607=CARTESIAN_POINT('Origin',(0.331856371369202,1.09142177001972,0.6));
#16608=CARTESIAN_POINT('Origin',(10.4681436286308,1.08420482079361,0.6));
#16609=CARTESIAN_POINT('Origin',(10.4681436276939,1.08420482084454,0.6));
#16610=CARTESIAN_POINT('',(10.5680065821063,1.08420482079361,0.605233595624295));
#16611=CARTESIAN_POINT('Origin',(10.4681436286308,1.08420482079361,0.6));
#16612=CARTESIAN_POINT('Origin',(10.4681436286308,1.08420482079361,0.6));
#16613=CARTESIAN_POINT('Origin',(0.3318563713692,-1.09142177001972,0.6));
#16614=CARTESIAN_POINT('Origin',(0.331856371369201,-1.09142177001972,0.6));
#16615=CARTESIAN_POINT('Origin',(0.3318563713692,-1.09142177001972,0.6));
#16616=CARTESIAN_POINT('Origin',(0.3318563713692,-0.7,0.6));
#16617=CARTESIAN_POINT('Ctrl Pts',(0.2922895713475,-1.22266882276207,-0.00177864096060679));
#16618=CARTESIAN_POINT('Ctrl Pts',(0.302885944515497,-1.21209940820877,
0.200681988163859));
#16619=CARTESIAN_POINT('Ctrl Pts',(0.313482241236256,-1.20153021465708,
0.403142632212487));
#16620=CARTESIAN_POINT('Ctrl Pts',(0.324078460244491,-1.19096124572524,
0.605603291426262));
#16621=CARTESIAN_POINT('Ctrl Pts',(0.264022491930188,-1.22039553779506,
-0.000415890128406236));
#16622=CARTESIAN_POINT('Ctrl Pts',(0.274621881512248,-1.20982222712748,
0.202044379074236));
#16623=CARTESIAN_POINT('Ctrl Pts',(0.285221154833576,-1.19924944554801,
0.404504681968985));
#16624=CARTESIAN_POINT('Ctrl Pts',(0.29582042516239,-1.18867654001483,0.606964977361795));
#16625=CARTESIAN_POINT('Ctrl Pts',(0.216712469170969,-1.1940874043406,0.000690255297866666));
#16626=CARTESIAN_POINT('Ctrl Pts',(0.227319688237882,-1.18351239299796,
0.203150045648192));
#16627=CARTESIAN_POINT('Ctrl Pts',(0.237926932441998,-1.17293746916702,
0.405609838636422));
#16628=CARTESIAN_POINT('Ctrl Pts',(0.248534117816369,-1.1623628476683,0.608069650238703));
#16629=CARTESIAN_POINT('Ctrl Pts',(0.200219987929043,-1.14439035743082,
-0.00103956457010847));
#16630=CARTESIAN_POINT('Ctrl Pts',(0.210830491339948,-1.13382006821851,
0.201420337884579));
#16631=CARTESIAN_POINT('Ctrl Pts',(0.221440906577676,-1.12324995278282,
0.403880253819325));
#16632=CARTESIAN_POINT('Ctrl Pts',(0.232051411471599,-1.11268010558856,
0.606340179010355));
#16633=CARTESIAN_POINT('Ctrl Pts',(0.200161975173303,-1.12312592850316,
-0.00214651389202307));
#16634=CARTESIAN_POINT('Ctrl Pts',(0.210772455448684,-1.11255764422181,
0.200313510564959));
#16635=CARTESIAN_POINT('Ctrl Pts',(0.221382936352032,-1.1019895901204,0.402773547004277));
#16636=CARTESIAN_POINT('Ctrl Pts',(0.231993417893744,-1.09142177001972,
0.605233595624295));
#16637=CARTESIAN_POINT('Origin',(10.4681436286308,-1.08420482109828,0.6));
#16638=CARTESIAN_POINT('',(10.5680065821063,-1.08420482079361,0.605233595624295));
#16639=CARTESIAN_POINT('Origin',(10.4681436286308,-1.08420482099672,0.600000000000001));
#16640=CARTESIAN_POINT('Origin',(10.4681436286308,-1.08420482109828,0.6));
#16641=CARTESIAN_POINT('Origin',(10.4681436286308,0.7,0.6));
#16642=CARTESIAN_POINT('',(10.5680065821063,0.7,0.605233595624295));
#16643=CARTESIAN_POINT('Ctrl Pts',(10.599839982685,-1.11594741464673,-0.00218387205330164));
#16644=CARTESIAN_POINT('Ctrl Pts',(10.5892288496247,-1.10536637943871,0.200288608282177));
#16645=CARTESIAN_POINT('Ctrl Pts',(10.5786177161011,-1.0947855138519,0.402761097457634));
#16646=CARTESIAN_POINT('Ctrl Pts',(10.5680065821063,-1.08420482079362,0.605233595624295));
#16647=CARTESIAN_POINT('Ctrl Pts',(10.5997613205547,-1.14474784499259,-0.000682909193257743));
#16648=CARTESIAN_POINT('Ctrl Pts',(10.5891501209488,-1.13416481604349,0.201789447273867));
#16649=CARTESIAN_POINT('Ctrl Pts',(10.5785391399155,-1.12358205581644,0.404261829287571));
#16650=CARTESIAN_POINT('Ctrl Pts',(10.5679279386544,-1.11299934606825,0.606734202078189));
#16651=CARTESIAN_POINT('Ctrl Pts',(10.5764119435127,-1.19466846760808,0.000702210001053139));
#16652=CARTESIAN_POINT('Ctrl Pts',(10.5658041809617,-1.18408222297768,0.203174550667819));
#16653=CARTESIAN_POINT('Ctrl Pts',(10.5551963844732,-1.17349608774572,0.405646894856767));
#16654=CARTESIAN_POINT('Ctrl Pts',(10.544588659013,-1.16291012508165,0.608119251464957));
#16655=CARTESIAN_POINT('Ctrl Pts',(10.5269342003857,-1.21442651155969,-0.000858270497959616));
#16656=CARTESIAN_POINT('Ctrl Pts',(10.5163317654776,-1.20384274018949,0.201614467507756));
#16657=CARTESIAN_POINT('Ctrl Pts',(10.5057293269973,-1.1932591813998,0.404087216090532));
#16658=CARTESIAN_POINT('Ctrl Pts',(10.4951269905998,-1.18267571840064,0.606559974437339));
#16659=CARTESIAN_POINT('Ctrl Pts',(10.5053655128635,-1.21565094114741,-0.0019246498908503));
#16660=CARTESIAN_POINT('Ctrl Pts',(10.4947646468921,-1.20506932615592,0.200548282383137));
#16661=CARTESIAN_POINT('Ctrl Pts',(10.4841638390504,-1.19448787589602,0.403021225840181));
#16662=CARTESIAN_POINT('Ctrl Pts',(10.4735630903435,-1.18390659316268,0.605494180667945));
#16663=CARTESIAN_POINT('Ctrl Pts',(10.5997255308004,-1.11583328740478,1.02782365951626E-16));
#16664=CARTESIAN_POINT('Ctrl Pts',(10.589152548365,-1.10529029582828,0.201744523047832));
#16665=CARTESIAN_POINT('Ctrl Pts',(10.5785795654695,-1.09474747266587,0.40348905487273));
#16666=CARTESIAN_POINT('Ctrl Pts',(10.5680065821063,-1.08420482079362,0.605233595624295));
#16667=CARTESIAN_POINT('Ctrl Pts',(10.5053638082297,1.21564923960921,-0.0018920919656423));
#16668=CARTESIAN_POINT('Ctrl Pts',(10.4947635104759,1.20506819181477,0.200569987667808));
#16669=CARTESIAN_POINT('Ctrl Pts',(10.4841632708454,1.19448730873444,0.403032078483127));
#16670=CARTESIAN_POINT('Ctrl Pts',(10.4735630903435,1.18390659316268,0.605494180667945));
#16671=CARTESIAN_POINT('Ctrl Pts',(10.5341220579192,1.21401666636749,-0.000470252816738081));
#16672=CARTESIAN_POINT('Ctrl Pts',(10.5235196325477,1.20343268662274,0.201991562854702));
#16673=CARTESIAN_POINT('Ctrl Pts',(10.5129172908767,1.19284910679518,0.404453403808947));
#16674=CARTESIAN_POINT('Ctrl Pts',(10.5023149573519,1.18226542681329,0.606915239027137));
#16675=CARTESIAN_POINT('Ctrl Pts',(10.5827170203615,1.18801090922716,0.000717463067903341));
#16676=CARTESIAN_POINT('Ctrl Pts',(10.5721088691741,1.17742555398174,0.203178921531494));
#16677=CARTESIAN_POINT('Ctrl Pts',(10.5615007184277,1.16684027916303,0.405640383775807));
#16678=CARTESIAN_POINT('Ctrl Pts',(10.5508925935528,1.15625520969485,0.60810185787831));
#16679=CARTESIAN_POINT('Ctrl Pts',(10.5997792798033,1.13754603572512,-0.00102559206997387));
#16680=CARTESIAN_POINT('Ctrl Pts',(10.5891686973038,1.12696411138589,0.201435946515793));
#16681=CARTESIAN_POINT('Ctrl Pts',(10.5785581831385,1.11638231376635,0.40389749513889));
#16682=CARTESIAN_POINT('Ctrl Pts',(10.5679475995174,1.10580071474959,0.606359050464716));
#16683=CARTESIAN_POINT('Ctrl Pts',(10.5998382764002,1.11594571320176,-0.00215131420076595));
#16684=CARTESIAN_POINT('Ctrl Pts',(10.5892277121014,1.10536524516024,0.200310313518148));
#16685=CARTESIAN_POINT('Ctrl Pts',(10.5786171473394,1.09478494672192,0.402771950076102));
#16686=CARTESIAN_POINT('Ctrl Pts',(10.5680065821063,1.08420482079361,0.605233595624295));
#16687=CARTESIAN_POINT('Ctrl Pts',(10.5680065821063,1.08420482079361,0.605233595624295));
#16688=CARTESIAN_POINT('Ctrl Pts',(10.5785795654695,1.09474747266587,0.40348905487273));
#16689=CARTESIAN_POINT('Ctrl Pts',(10.589152548365,1.10529029582828,0.201744523047831));
#16690=CARTESIAN_POINT('Ctrl Pts',(10.5997255308004,1.11583328740478,1.07661275727811E-16));
#16691=CARTESIAN_POINT('Ctrl Pts',(10.1947388861048,1.09885088260187,0.7));
#16692=CARTESIAN_POINT('Ctrl Pts',(10.285877616441,1.09404209584202,0.7));
#16693=CARTESIAN_POINT('Ctrl Pts',(10.3770124662346,1.0891584122264,0.7));
#16694=CARTESIAN_POINT('Ctrl Pts',(10.4681436286308,1.08420482079361,0.7));
#16695=CARTESIAN_POINT('Ctrl Pts',(10.196260416419,1.12768774893097,0.700000000000001));
#16696=CARTESIAN_POINT('Ctrl Pts',(10.2874149314686,1.12287675076168,0.699999949550842));
#16697=CARTESIAN_POINT('Ctrl Pts',(10.3785648662465,1.11799094453753,0.700000051218742));
#16698=CARTESIAN_POINT('Ctrl Pts',(10.4697107510168,1.11303515260326,0.7));
#16699=CARTESIAN_POINT('Ctrl Pts',(10.1988975981852,1.17766904563614,0.67669140632491));
#16700=CARTESIAN_POINT('Ctrl Pts',(10.2900793016129,1.17285439035486,0.676693724638983));
#16701=CARTESIAN_POINT('Ctrl Pts',(10.3812557252598,1.16796482352885,0.676696026813929));
#16702=CARTESIAN_POINT('Ctrl Pts',(10.4724269697127,1.16300539549315,0.676698381019544));
#16703=CARTESIAN_POINT('Ctrl Pts',(10.1999375452555,1.19737868557977,0.627098033786781));
#16704=CARTESIAN_POINT('Ctrl Pts',(10.2911301919381,1.19256517083271,0.627104033151799));
#16705=CARTESIAN_POINT('Ctrl Pts',(10.382317043787,1.18767684023183,0.627110048826767));
#16706=CARTESIAN_POINT('Ctrl Pts',(10.4734985149421,1.18271860027509,0.627116141711795));
#16707=CARTESIAN_POINT('Ctrl Pts',(10.1999999975038,1.19856231440453,0.605472757505366));
#16708=CARTESIAN_POINT('Ctrl Pts',(10.2911933328565,1.19375025772558,0.605479840815741));
#16709=CARTESIAN_POINT('Ctrl Pts',(10.3823809652617,1.18886335120032,0.605486986548286));
#16710=CARTESIAN_POINT('Ctrl Pts',(10.4735630903435,1.18390659316268,0.605494180667944));
#16711=CARTESIAN_POINT('Ctrl Pts',(0.200159601751749,1.12312829248604,-0.00219180147311912));
#16712=CARTESIAN_POINT('Ctrl Pts',(0.210770873167554,1.11255922017607,0.200283318842441));
#16713=CARTESIAN_POINT('Ctrl Pts',(0.221382145211419,1.10199037808008,0.402758451142111));
#16714=CARTESIAN_POINT('Ctrl Pts',(0.231993417893744,1.09142177001972,0.605233595624295));
#16715=CARTESIAN_POINT('Ctrl Pts',(0.200236952094631,1.15148086499205,-0.000715869007730825));
#16716=CARTESIAN_POINT('Ctrl Pts',(0.210848310847714,1.14090905181173,0.201759082033021));
#16717=CARTESIAN_POINT('Ctrl Pts',(0.221459381762758,1.13033759660317,0.404234066901971));
#16718=CARTESIAN_POINT('Ctrl Pts',(0.232070742664217,1.11976621744484,0.606709040139042));
#16719=CARTESIAN_POINT('Ctrl Pts',(0.222806696702742,1.20067708175657,0.000669311976984441));
#16720=CARTESIAN_POINT('Ctrl Pts',(0.233413416075889,1.19010082554658,0.203144236955742));
#16721=CARTESIAN_POINT('Ctrl Pts',(0.244020198555212,1.17952469009474,0.405619164345205));
#16722=CARTESIAN_POINT('Ctrl Pts',(0.254626870458834,1.16894881850735,0.608094110943904));
#16723=CARTESIAN_POINT('Ctrl Pts',(0.271086891015657,1.22096622390789,-0.000801865493577694));
#16724=CARTESIAN_POINT('Ctrl Pts',(0.281686280594249,1.21039315447922,0.201673594461172));
#16725=CARTESIAN_POINT('Ctrl Pts',(0.292285672737775,1.1998203699977,0.404149068703718));
#16726=CARTESIAN_POINT('Ctrl Pts',(0.302884933932915,1.18924771644243,0.606624555877912));
#16727=CARTESIAN_POINT('Ctrl Pts',(0.292287201081515,1.22267118699778,-0.00182392867695869));
#16728=CARTESIAN_POINT('Ctrl Pts',(0.302884364349574,1.21210098433295,0.200651796350731));
#16729=CARTESIAN_POINT('Ctrl Pts',(0.313481451159089,1.20153100270242,0.403127536304793));
#16730=CARTESIAN_POINT('Ctrl Pts',(0.324078460244491,1.19096124572524,0.605603291426262));
#16731=CARTESIAN_POINT('Origin',(10.6002740930491,1.4,-0.0104671912485891));
#16732=CARTESIAN_POINT('Origin',(0.331856371369202,1.09142177001972,0.6));
#16733=CARTESIAN_POINT('',(0.3318563713692,1.09142177001972,0.9));
#16734=CARTESIAN_POINT('',(0.0322675109428288,1.09142177001972,0.615700786872883));
#16735=CARTESIAN_POINT('Origin',(0.3318563713692,1.09142177001972,0.6));
#16736=CARTESIAN_POINT('',(0.308522637995069,1.39004019713626,0.616809874278785));
#16737=CARTESIAN_POINT('Origin',(0.331856371369202,1.09142177001972,0.6));
#16738=CARTESIAN_POINT('Origin',(0.331856371369201,1.09142177001972,0.6));
#16739=CARTESIAN_POINT('Origin',(10.4681436286308,1.08420482079361,0.6));
#16740=CARTESIAN_POINT('',(10.4681436286308,1.08420482109828,0.9));
#16741=CARTESIAN_POINT('',(10.4844020137689,1.3833101379008,0.616482542003833));
#16742=CARTESIAN_POINT('Origin',(10.4681436258201,1.08420482094639,0.6));
#16743=CARTESIAN_POINT('',(10.7677324890572,1.08420482079361,0.615700786872884));
#16744=CARTESIAN_POINT('Origin',(10.4681436286308,1.08420482079361,0.6));
#16745=CARTESIAN_POINT('Origin',(10.4681436286308,1.08420482079362,0.6));
#16746=CARTESIAN_POINT('Origin',(0.3318563713692,-1.09142177001972,0.6));
#16747=CARTESIAN_POINT('',(0.3318563713692,-1.09142177001972,0.9));
#16748=CARTESIAN_POINT('',(0.308522637995069,-1.39004019713626,0.616809874278785));
#16749=CARTESIAN_POINT('Origin',(0.3318563713692,-1.09142177001972,0.6));
#16750=CARTESIAN_POINT('',(0.0322675109428289,-1.09142177001972,0.615700786872884));
#16751=CARTESIAN_POINT('Origin',(0.3318563713692,-1.09142177001972,0.6));
#16752=CARTESIAN_POINT('Origin',(0.331856371369201,-1.09142177001972,0.6));
#16753=CARTESIAN_POINT('Origin',(0.3318563713692,-0.7,0.6));
#16754=CARTESIAN_POINT('',(0.0322675109428288,-0.7,0.615700786872883));
#16755=CARTESIAN_POINT('',(0.3318563713692,-0.7,0.9));
#16756=CARTESIAN_POINT('Ctrl Pts',(0.276048389810261,-1.42252533450788,
-0.00533608639730399));
#16757=CARTESIAN_POINT('Ctrl Pts',(0.28687338241706,-1.4116967417008,0.202045878554724));
#16758=CARTESIAN_POINT('Ctrl Pts',(0.297698133178874,-1.40086836142621,
0.409427865329919));
#16759=CARTESIAN_POINT('Ctrl Pts',(0.308522637995069,-1.39004019713626,
0.616809874278785));
#16760=CARTESIAN_POINT('Ctrl Pts',(0.191246496057484,-1.41570630783033,
-0.00124775669238285));
#16761=CARTESIAN_POINT('Ctrl Pts',(0.202080757839133,-1.40486573978029,
0.206133102090467));
#16762=CARTESIAN_POINT('Ctrl Pts',(0.212914648880055,-1.39402634701096,
0.413514041581016));
#16763=CARTESIAN_POINT('Ctrl Pts',(0.223748532748767,-1.38318608000504,
0.620894932085382));
#16764=CARTESIAN_POINT('Ctrl Pts',(0.0492682973509243,-1.33685850703924,
0.00207719607616587));
#16765=CARTESIAN_POINT('Ctrl Pts',(0.0601266125734448,-1.32601270457081,
0.209456583216085));
#16766=CARTESIAN_POINT('Ctrl Pts',(0.0709850253737815,-1.3151666447344,
0.416835949794532));
#16767=CARTESIAN_POINT('Ctrl Pts',(0.0818432319483421,-1.30432109509162,
0.624215353109623));
#16768=CARTESIAN_POINT('Ctrl Pts',(-0.000163444061205068,-1.18769013309795,
-0.00311869847265479));
#16769=CARTESIAN_POINT('Ctrl Pts',(0.0107049555364969,-1.17685886333949,
0.204261034729081));
#16770=CARTESIAN_POINT('Ctrl Pts',(0.0215730900970294,-1.16602762920277,
0.411640782964944));
#16771=CARTESIAN_POINT('Ctrl Pts',(0.0324414916763936,-1.15519677672624,
0.619020537031064));
#16772=CARTESIAN_POINT('Ctrl Pts',(-0.00033748371827097,-1.12389640457412,
-0.0064395729582146));
#16773=CARTESIAN_POINT('Ctrl Pts',(0.0105308471731094,-1.11307128361434,
0.200940534347673));
#16774=CARTESIAN_POINT('Ctrl Pts',(0.0213991787230862,-1.10224640406117,
0.408320654220332));
#16775=CARTESIAN_POINT('Ctrl Pts',(0.0322675109428289,-1.09142177001972,
0.615700786872884));
#16776=CARTESIAN_POINT('Ctrl Pts',(0.27632692456468,-1.42224670711126,5.13911829758129E-17));
#16777=CARTESIAN_POINT('Ctrl Pts',(0.287059068122268,-1.41151099373342,
0.20560326985903));
#16778=CARTESIAN_POINT('Ctrl Pts',(0.297790973931072,-1.40077548928706,
0.411206561171438));
#16779=CARTESIAN_POINT('Ctrl Pts',(0.308522637995069,-1.39004019713626,
0.616809874278785));
#16780=CARTESIAN_POINT('Ctrl Pts',(0.0322675109428289,-1.09142177001972,
0.615700786872884));
#16781=CARTESIAN_POINT('Ctrl Pts',(0.0215116733095221,-1.10213436178043,
0.410467178800746));
#16782=CARTESIAN_POINT('Ctrl Pts',(0.0107558363321879,-1.11284719399673,
0.205233583245308));
#16783=CARTESIAN_POINT('Ctrl Pts',(1.76901136968166E-16,-1.12356026268968,
-7.45931094670027E-17));
#16784=CARTESIAN_POINT('Origin',(10.4681436286308,-1.08420482109828,0.6));
#16785=CARTESIAN_POINT('',(10.7677324890572,-1.08420482079361,0.615700786872884));
#16786=CARTESIAN_POINT('',(10.4844020137689,-1.3833101379008,0.616482542003833));
#16787=CARTESIAN_POINT('Origin',(10.4681436286308,-1.08420482079361,0.600000000000001));
#16788=CARTESIAN_POINT('',(10.4681436258201,-1.08420482094639,0.9));
#16789=CARTESIAN_POINT('Origin',(10.4681436286308,-1.08420482109828,0.6));
#16790=CARTESIAN_POINT('Origin',(10.4681436286308,-1.08420482079361,0.6));
#16791=CARTESIAN_POINT('Origin',(10.4681436286308,0.7,0.6));
#16792=CARTESIAN_POINT('',(10.7677324890572,0.7,0.615700786872884));
#16793=CARTESIAN_POINT('',(10.4681436286308,0.7,0.9));
#16794=CARTESIAN_POINT('Ctrl Pts',(10.4681436286308,-1.08420482079361,0.9));
#16795=CARTESIAN_POINT('Ctrl Pts',(9.02115959826777,-1.16285813221549,0.9));
#16796=CARTESIAN_POINT('Ctrl Pts',(5.64262097844114,-1.30550334054488,0.9));
#16797=CARTESIAN_POINT('Ctrl Pts',(2.25816172369615,-1.24194126716656,0.9));
#16798=CARTESIAN_POINT('Ctrl Pts',(0.331856371369198,-1.09142177001972,
0.9));
#16799=CARTESIAN_POINT('Ctrl Pts',(10.4728449957889,-1.17069581622255,0.9));
#16800=CARTESIAN_POINT('Ctrl Pts',(9.02515960257209,-1.24945398332951,0.900002463983243));
#16801=CARTESIAN_POINT('Ctrl Pts',(5.64406008560805,-1.39235654229312,0.899995181674544));
#16802=CARTESIAN_POINT('Ctrl Pts',(2.25481214769604,-1.3286896492945,0.900006992415263));
#16803=CARTESIAN_POINT('Ctrl Pts',(0.325113511056834,-1.17771496230318,
0.9));
#16804=CARTESIAN_POINT('Ctrl Pts',(10.4809942371438,-1.32061731204901,0.830050158657121));
#16805=CARTESIAN_POINT('Ctrl Pts',(9.03210079995546,-1.3995487214628,0.829938185878055));
#16806=CARTESIAN_POINT('Ctrl Pts',(5.64656962219688,-1.54290142969263,0.82970437227026));
#16807=CARTESIAN_POINT('Ctrl Pts',(2.24896854757963,-1.47903552984056,0.829838703712927));
#16808=CARTESIAN_POINT('Ctrl Pts',(0.313425270489114,-1.32729771265557,
0.830156825336737));
#16809=CARTESIAN_POINT('Ctrl Pts',(10.4842082875648,-1.37974615923803,0.681348425135383));
#16810=CARTESIAN_POINT('Ctrl Pts',(9.03482793853036,-1.45862084618981,0.681058092399338));
#16811=CARTESIAN_POINT('Ctrl Pts',(5.64753778607331,-1.60187726023264,0.68045297450285));
#16812=CARTESIAN_POINT('Ctrl Pts',(2.24670449952385,-1.53809938127555,0.680799765935021));
#16813=CARTESIAN_POINT('Ctrl Pts',(0.308806004580392,-1.38641375285276,
0.681625057916928));
#16814=CARTESIAN_POINT('Ctrl Pts',(10.4844020137689,-1.3833101379008,0.616482542003833));
#16815=CARTESIAN_POINT('Ctrl Pts',(9.03499042108131,-1.46211428773623,0.616139856494792));
#16816=CARTESIAN_POINT('Ctrl Pts',(5.64759185703765,-1.60522711936681,0.615422163720642));
#16817=CARTESIAN_POINT('Ctrl Pts',(2.24657199659733,-1.54153220865049,0.615835494619844));
#16818=CARTESIAN_POINT('Ctrl Pts',(0.308522637995066,-1.39004019713626,
0.616809874278785));
#16819=CARTESIAN_POINT('Ctrl Pts',(0.308522637995066,-1.39004019713626,
0.616809874278785));
#16820=CARTESIAN_POINT('Ctrl Pts',(2.24657199659733,-1.54153220865049,0.615835494619844));
#16821=CARTESIAN_POINT('Ctrl Pts',(5.64759185703765,-1.60522711936681,0.615422163720642));
#16822=CARTESIAN_POINT('Ctrl Pts',(9.03499042108131,-1.46211428773623,0.616139856494792));
#16823=CARTESIAN_POINT('Ctrl Pts',(10.4844020137689,-1.3833101379008,0.616482542003833));
#16824=CARTESIAN_POINT('Ctrl Pts',(10.4681436258201,-1.08420482094639,0.900000000000001));
#16825=CARTESIAN_POINT('Ctrl Pts',(9.02115959639274,-1.16285813229465,0.9));
#16826=CARTESIAN_POINT('Ctrl Pts',(5.64262097750198,-1.30550334052724,0.9));
#16827=CARTESIAN_POINT('Ctrl Pts',(2.25816172369615,-1.24194126716656,0.9));
#16828=CARTESIAN_POINT('Ctrl Pts',(0.331856371369198,-1.09142177001972,
0.9));
#16829=CARTESIAN_POINT('Ctrl Pts',(10.8003433549902,-1.11672267507076,-0.00655160349952438));
#16830=CARTESIAN_POINT('Ctrl Pts',(10.7894730668347,-1.10588321133639,0.200865850630566));
#16831=CARTESIAN_POINT('Ctrl Pts',(10.7786027781932,-1.09504392553578,0.408283314033857));
#16832=CARTESIAN_POINT('Ctrl Pts',(10.7677324890572,-1.08420482079361,0.615700786872885));
#16833=CARTESIAN_POINT('Ctrl Pts',(10.8001073672393,-1.20312439623403,-0.00204868896805508));
#16834=CARTESIAN_POINT('Ctrl Pts',(10.7892368724076,-1.19227880391739,0.205368384315645));
#16835=CARTESIAN_POINT('Ctrl Pts',(10.7783670568079,-1.18143370221047,0.41278551899075));
#16836=CARTESIAN_POINT('Ctrl Pts',(10.7674965587017,-1.17058839661753,0.620202606234566));
#16837=CARTESIAN_POINT('Ctrl Pts',(10.7300137544668,-1.35289768637741,0.00210488808650419));
#16838=CARTESIAN_POINT('Ctrl Pts',(10.7191538066016,-1.34204221082848,0.209521911971666));
#16839=CARTESIAN_POINT('Ctrl Pts',(10.7082938463195,-1.33118673671862,0.416938933985702));
#16840=CARTESIAN_POINT('Ctrl Pts',(10.6974340169938,-1.32033143065575,0.624355970618915));
#16841=CARTESIAN_POINT('Ctrl Pts',(10.5816241002662,-1.4121605627967,-0.00257485550010117));
#16842=CARTESIAN_POINT('Ctrl Pts',(10.5707805459565,-1.4013126969686,0.204843391064434));
#16843=CARTESIAN_POINT('Ctrl Pts',(10.5599369567012,-1.39046512672587,0.412261650129749));
#16844=CARTESIAN_POINT('Ctrl Pts',(10.5490937145378,-1.37961751361469,0.619679923312015));
#16845=CARTESIAN_POINT('Ctrl Pts',(10.5169176890673,-1.41583338198674,-0.00577403633861717));
#16846=CARTESIAN_POINT('Ctrl Pts',(10.5060789456421,-1.40499213715574,0.201644806368331));
#16847=CARTESIAN_POINT('Ctrl Pts',(10.4952403861233,-1.39415105487295,0.40906366572247));
#16848=CARTESIAN_POINT('Ctrl Pts',(10.4844020137689,-1.3833101379008,0.616482542003833));
#16849=CARTESIAN_POINT('Ctrl Pts',(10.8,-1.11638029377732,-2.51534904016637E-17));
#16850=CARTESIAN_POINT('Ctrl Pts',(10.7892441634977,-1.10565496086826,0.205233586491178));
#16851=CARTESIAN_POINT('Ctrl Pts',(10.7784883265195,-1.09492980219801,0.410467182062988));
#16852=CARTESIAN_POINT('Ctrl Pts',(10.7677324890572,-1.08420482079361,0.615700786872885));
#16853=CARTESIAN_POINT('Ctrl Pts',(10.4844020137689,-1.3833101379008,0.616482542003833));
#16854=CARTESIAN_POINT('Ctrl Pts',(10.4951398148107,-1.39405045994841,0.410988344812119));
#16855=CARTESIAN_POINT('Ctrl Pts',(10.5058777995597,-1.40479094425298,0.205494164234945));
#16856=CARTESIAN_POINT('Ctrl Pts',(10.5166159648474,-1.4155315881283,-2.5652223401007E-16));
#16857=CARTESIAN_POINT('Ctrl Pts',(10.5169125872774,1.41582827901939,-0.0056764044152427));
#16858=CARTESIAN_POINT('Ctrl Pts',(10.5060755445066,1.40498873522851,0.20170989432247));
#16859=CARTESIAN_POINT('Ctrl Pts',(10.4952386855848,1.39414935393528,0.409096209702196));
#16860=CARTESIAN_POINT('Ctrl Pts',(10.4844020137689,1.3833101379008,0.616482542003833));
#16861=CARTESIAN_POINT('Ctrl Pts',(10.6031877991504,1.41093118264609,-0.00141083033817288));
#16862=CARTESIAN_POINT('Ctrl Pts',(10.5923442181457,1.40008262840665,0.205974657203891));
#16863=CARTESIAN_POINT('Ctrl Pts',(10.5815009048179,1.38923496752292,0.413360205434192));
#16864=CARTESIAN_POINT('Ctrl Pts',(10.5706576147941,1.37838663885266,0.62074571708141));
#16865=CARTESIAN_POINT('Ctrl Pts',(10.7489822201969,1.33286898269122,0.00215046584238339));
#16866=CARTESIAN_POINT('Ctrl Pts',(10.7381210493968,1.32201618867047,0.209534855263179));
#16867=CARTESIAN_POINT('Ctrl Pts',(10.7272598662103,1.31116338896628,0.416919242515175));
#16868=CARTESIAN_POINT('Ctrl Pts',(10.716398780155,1.30031077634578,0.624303643734563));
#16869=CARTESIAN_POINT('Ctrl Pts',(10.8001612475457,1.18151886169146,-0.00307678645922502));
#16870=CARTESIAN_POINT('Ctrl Pts',(10.7892926103682,1.17067663552019,0.20430785074418));
#16871=CARTESIAN_POINT('Ctrl Pts',(10.7784241800195,1.15983442267521,0.41169249890798));
#16872=CARTESIAN_POINT('Ctrl Pts',(10.7675555412906,1.14899250266155,0.619077151394146));
#16873=CARTESIAN_POINT('Ctrl Pts',(10.8003382383521,1.11671757294177,-0.00645397222975308));
#16874=CARTESIAN_POINT('Ctrl Pts',(10.7894696557425,1.1058798099729,0.200930938146656));
#16875=CARTESIAN_POINT('Ctrl Pts',(10.778601072647,1.09504222488243,0.408315857793383));
#16876=CARTESIAN_POINT('Ctrl Pts',(10.7677324890572,1.08420482079361,0.615700786872884));
#16877=CARTESIAN_POINT('Ctrl Pts',(10.5166159648474,1.4155315881283,3.37837396946483E-16));
#16878=CARTESIAN_POINT('Ctrl Pts',(10.5058777995597,1.40479094425298,0.205494164234944));
#16879=CARTESIAN_POINT('Ctrl Pts',(10.4951398148107,1.39405045994841,0.41098834481212));
#16880=CARTESIAN_POINT('Ctrl Pts',(10.4844020137689,1.3833101379008,0.616482542003833));
#16881=CARTESIAN_POINT('Ctrl Pts',(10.7677324890572,1.08420482079361,0.615700786872884));
#16882=CARTESIAN_POINT('Ctrl Pts',(10.7784883265195,1.09492980219801,0.410467182062988));
#16883=CARTESIAN_POINT('Ctrl Pts',(10.7892441634977,1.10565496086826,0.205233586491177));
#16884=CARTESIAN_POINT('Ctrl Pts',(10.8,1.11638029377732,-4.7271214720368E-17));
#16885=CARTESIAN_POINT('Ctrl Pts',(0.3318563713692,1.09142177001972,0.9));
#16886=CARTESIAN_POINT('Ctrl Pts',(1.77658538561441,1.20431139287985,0.9));
#16887=CARTESIAN_POINT('Ctrl Pts',(5.15852145577913,1.31798734362749,0.900000000000001));
#16888=CARTESIAN_POINT('Ctrl Pts',(8.53883158814675,1.18907590268945,0.9));
#16889=CARTESIAN_POINT('Ctrl Pts',(10.4681436286308,1.08420482079361,0.9));
#16890=CARTESIAN_POINT('Ctrl Pts',(0.325113511056836,1.17771496230318,0.9));
#16891=CARTESIAN_POINT('Ctrl Pts',(1.77238748853623,1.29094597754667,0.900005244311447));
#16892=CARTESIAN_POINT('Ctrl Pts',(5.15940689953628,1.40489117512763,0.899995532233175));
#16893=CARTESIAN_POINT('Ctrl Pts',(8.54259780483314,1.2757067056985,0.90000328531099));
#16894=CARTESIAN_POINT('Ctrl Pts',(10.4728449957889,1.17069581622255,0.9));
#16895=CARTESIAN_POINT('Ctrl Pts',(0.313425270489116,1.32729771265557,0.830156825336737));
#16896=CARTESIAN_POINT('Ctrl Pts',(1.76508272830699,1.44110107554431,0.829918234118879));
#16897=CARTESIAN_POINT('Ctrl Pts',(5.16095094050242,1.55552201031752,0.829677185710002));
#16898=CARTESIAN_POINT('Ctrl Pts',(8.54913632089268,1.4258591912674,0.829900861618366));
#16899=CARTESIAN_POINT('Ctrl Pts',(10.4809942371438,1.32061731204901,0.830050158657121));
#16900=CARTESIAN_POINT('Ctrl Pts',(0.308806004580394,1.38641375285276,0.681625057916928));
#16901=CARTESIAN_POINT('Ctrl Pts',(1.76222987578798,1.50017797416985,0.681006088930498));
#16902=CARTESIAN_POINT('Ctrl Pts',(5.16154986224672,1.61450132085358,0.68038246417749));
#16903=CARTESIAN_POINT('Ctrl Pts',(8.55170115551887,1.48491240850707,0.680961314820656));
#16904=CARTESIAN_POINT('Ctrl Pts',(10.4842082875648,1.37974615923803,0.681348425135383));
#16905=CARTESIAN_POINT('Ctrl Pts',(0.308522637995068,1.39004019713626,0.616809874278785));
#16906=CARTESIAN_POINT('Ctrl Pts',(1.76205965694675,1.50365920577193,0.616079089534579));
#16907=CARTESIAN_POINT('Ctrl Pts',(5.16158497046229,1.61783515152865,0.615338844765104));
#16908=CARTESIAN_POINT('Ctrl Pts',(8.55185322351876,1.48838233768137,0.616025627991778));
#16909=CARTESIAN_POINT('Ctrl Pts',(10.4844020137689,1.3833101379008,0.616482542003833));
#16910=CARTESIAN_POINT('Ctrl Pts',(10.4844020137689,1.3833101379008,0.616482542003833));
#16911=CARTESIAN_POINT('Ctrl Pts',(8.55185322351876,1.48838233768137,0.616025627991778));
#16912=CARTESIAN_POINT('Ctrl Pts',(5.16158497046229,1.61783515152865,0.615338844765104));
#16913=CARTESIAN_POINT('Ctrl Pts',(1.76205965694675,1.50365920577193,0.616079089534579));
#16914=CARTESIAN_POINT('Ctrl Pts',(0.308522637995068,1.39004019713626,0.616809874278785));
#16915=CARTESIAN_POINT('Ctrl Pts',(0.3318563713692,1.09142177001972,0.9));
#16916=CARTESIAN_POINT('Ctrl Pts',(1.77658538561441,1.20431139287985,0.9));
#16917=CARTESIAN_POINT('Ctrl Pts',(5.15852145577913,1.31798734362749,0.900000000000001));
#16918=CARTESIAN_POINT('Ctrl Pts',(8.53883158814675,1.18907590268945,0.9));
#16919=CARTESIAN_POINT('Ctrl Pts',(10.4681436286308,1.08420482079361,0.9));
#16920=CARTESIAN_POINT('Ctrl Pts',(-0.000344602063817145,1.12390349461883,
-0.00657539908256866));
#16921=CARTESIAN_POINT('Ctrl Pts',(0.0105261016091243,1.11307601020539,
0.200849983592616));
#16922=CARTESIAN_POINT('Ctrl Pts',(0.0213968059409475,1.10224876730309,
0.408275378840013));
#16923=CARTESIAN_POINT('Ctrl Pts',(0.0322675109428289,1.09142177001972,
0.615700786872884));
#16924=CARTESIAN_POINT('Ctrl Pts',(-0.000112549170678945,1.2089618047365,
-0.00214756610981592));
#16925=CARTESIAN_POINT('Ctrl Pts',(0.0107584275574203,1.19812589474889,
0.205277296000037));
#16926=CARTESIAN_POINT('Ctrl Pts',(0.021628504370896,1.18729063034778,0.412702239156743));
#16927=CARTESIAN_POINT('Ctrl Pts',(0.0324994852542487,1.17645511229507,
0.620127120417125));
#16928=CARTESIAN_POINT('Ctrl Pts',(0.0675181008536004,1.35659180908255,
0.00201426213057289));
#16929=CARTESIAN_POINT('Ctrl Pts',(0.0783748317004002,1.34574224493831,
0.20943904356877));
#16930=CARTESIAN_POINT('Ctrl Pts',(0.0892318011706237,1.33489254525337,
0.416863803530356));
#16931=CARTESIAN_POINT('Ctrl Pts',(0.100088380073201,1.32404321751407,0.624288602298589));
#16932=CARTESIAN_POINT('Ctrl Pts',(0.212439875011655,1.41741816253371,-0.00240566592686199));
#16933=CARTESIAN_POINT('Ctrl Pts',(0.223274062163905,1.40657840226088,0.20502076110302));
#16934=CARTESIAN_POINT('Ctrl Pts',(0.234108278795672,1.39573903465802,0.412447205628077));
#16935=CARTESIAN_POINT('Ctrl Pts',(0.244942059060342,1.38489960928785,0.619873667633733));
#16936=CARTESIAN_POINT('Ctrl Pts',(0.276041299849618,1.42253242682652,-0.00547191373834488));
#16937=CARTESIAN_POINT('Ctrl Pts',(0.286868655882245,1.41170146982041,0.201955326984501));
#16938=CARTESIAN_POINT('Ctrl Pts',(0.297695769965166,1.40087072543886,0.409382589539965));
#16939=CARTESIAN_POINT('Ctrl Pts',(0.308522637995069,1.39004019713626,0.616809874278785));
#16940=CARTESIAN_POINT('Ctrl Pts',(2.26869304592592E-17,1.12356026268968,
-3.16587034365767E-17));
#16941=CARTESIAN_POINT('Ctrl Pts',(0.0107558363321878,1.11284719399672,
0.205233583245308));
#16942=CARTESIAN_POINT('Ctrl Pts',(0.0215116733095221,1.10213436178043,
0.410467178800746));
#16943=CARTESIAN_POINT('Ctrl Pts',(0.0322675109428289,1.09142177001972,
0.615700786872884));
#16944=CARTESIAN_POINT('Ctrl Pts',(0.308522637995069,1.39004019713626,0.616809874278785));
#16945=CARTESIAN_POINT('Ctrl Pts',(0.297790973931072,1.40077548928706,0.411206561171438));
#16946=CARTESIAN_POINT('Ctrl Pts',(0.287059068122271,1.41151099373341,0.205603269859031));
#16947=CARTESIAN_POINT('Ctrl Pts',(0.276326924564681,1.42224670711126,-2.68882138776405E-16));
#16948=CARTESIAN_POINT('Ctrl Pts',(10.5166159648474,-1.4155315881283,0.));
#16949=CARTESIAN_POINT('Ctrl Pts',(10.5064062201588,-1.40475637621136,0.205603291426271));
#16950=CARTESIAN_POINT('Ctrl Pts',(10.4961964754701,-1.39398116429443,0.411206582852543));
#16951=CARTESIAN_POINT('Ctrl Pts',(10.4859867307814,-1.38320595237749,0.616809874278814));
#16952=CARTESIAN_POINT('Ctrl Pts',(7.10318628475318,-1.599994843061,0.));
#16953=CARTESIAN_POINT('Ctrl Pts',(7.09978773046573,-1.58921963114407,0.205603291426271));
#16954=CARTESIAN_POINT('Ctrl Pts',(7.09638917617828,-1.57844441922713,0.411206582852543));
#16955=CARTESIAN_POINT('Ctrl Pts',(7.09299062189083,-1.5676692073102,0.616809874278814));
#16956=CARTESIAN_POINT('Ctrl Pts',(3.68975660465893,-1.68747752195839,0.));
#16957=CARTESIAN_POINT('Ctrl Pts',(3.69316924077269,-1.67670231004145,0.205603291426272));
#16958=CARTESIAN_POINT('Ctrl Pts',(3.69658187688646,-1.66592709812452,0.411206582852543));
#16959=CARTESIAN_POINT('Ctrl Pts',(3.69999451300023,-1.65515188620758,0.616809874278814));
#16960=CARTESIAN_POINT('Ctrl Pts',(0.276326924564679,-1.42224670711126,
0.));
#16961=CARTESIAN_POINT('Ctrl Pts',(0.286550751079662,-1.41147149519433,
0.205603291426271));
#16962=CARTESIAN_POINT('Ctrl Pts',(0.296774577594646,-1.40069628327739,
0.411206582852543));
#16963=CARTESIAN_POINT('Ctrl Pts',(0.306998404109629,-1.38992107136046,
0.616809874278814));
#16964=CARTESIAN_POINT('Origin',(0.,-1.4,0.));
#16965=CARTESIAN_POINT('Origin',(5.4,-8.13935059369636E-18,0.9));
#16966=CARTESIAN_POINT('Ctrl Pts',(0.276326924564679,1.42224670711126,0.));
#16967=CARTESIAN_POINT('Ctrl Pts',(0.286550751079662,1.41147149519433,0.205603291426271));
#16968=CARTESIAN_POINT('Ctrl Pts',(0.296774577594645,1.40069628327739,0.411206582852543));
#16969=CARTESIAN_POINT('Ctrl Pts',(0.306998404109628,1.38992107136046,0.616809874278814));
#16970=CARTESIAN_POINT('Ctrl Pts',(3.68975660465893,1.68747752195839,0.));
#16971=CARTESIAN_POINT('Ctrl Pts',(3.6931692407727,1.67670231004145,0.205603291426271));
#16972=CARTESIAN_POINT('Ctrl Pts',(3.69658187688646,1.66592709812452,0.411206582852543));
#16973=CARTESIAN_POINT('Ctrl Pts',(3.69999451300023,1.65515188620758,0.616809874278814));
#16974=CARTESIAN_POINT('Ctrl Pts',(7.10318628475318,1.599994843061,0.));
#16975=CARTESIAN_POINT('Ctrl Pts',(7.09978773046573,1.58921963114407,0.205603291426271));
#16976=CARTESIAN_POINT('Ctrl Pts',(7.09638917617828,1.57844441922713,0.411206582852543));
#16977=CARTESIAN_POINT('Ctrl Pts',(7.09299062189083,1.5676692073102,0.616809874278814));
#16978=CARTESIAN_POINT('Ctrl Pts',(10.5166159648474,1.4155315881283,0.));
#16979=CARTESIAN_POINT('Ctrl Pts',(10.5064062201588,1.40475637621136,0.205603291426271));
#16980=CARTESIAN_POINT('Ctrl Pts',(10.4961964754701,1.39398116429443,0.411206582852543));
#16981=CARTESIAN_POINT('Ctrl Pts',(10.4859867307814,1.38320595237749,0.616809874278814));
#16982=CARTESIAN_POINT('Origin',(10.8,1.4,0.));
#24790=UNCERTAINTY_MEASURE_WITH_UNIT(LENGTH_MEASURE(0.001),#24810,
'DISTANCE_ACCURACY_VALUE',
'Maximum model space distance between geometric entities at asserted c
onnectivities');
#24796=UNCERTAINTY_MEASURE_WITH_UNIT(LENGTH_MEASURE(0.001),#24810,
'DISTANCE_ACCURACY_VALUE',
'Maximum model space distance between geometric entities at asserted c
onnectivities');
#24803=(
GEOMETRIC_REPRESENTATION_CONTEXT(3)
GLOBAL_UNCERTAINTY_ASSIGNED_CONTEXT((#24790))
GLOBAL_UNIT_ASSIGNED_CONTEXT((#24810,#24812,#24813))
REPRESENTATION_CONTEXT('','3D')
);
#24809=(
GEOMETRIC_REPRESENTATION_CONTEXT(3)
GLOBAL_UNCERTAINTY_ASSIGNED_CONTEXT((#24796))
GLOBAL_UNIT_ASSIGNED_CONTEXT((#24810,#24812,#24813))
REPRESENTATION_CONTEXT('','3D')
);
#24810=(
LENGTH_UNIT()
NAMED_UNIT(*)
SI_UNIT(.CENTI.,.METRE.)
);
#24812=(
NAMED_UNIT(*)
PLANE_ANGLE_UNIT()
SI_UNIT($,.RADIAN.)
);
#24813=(
NAMED_UNIT(*)
SI_UNIT($,.STERADIAN.)
SOLID_ANGLE_UNIT()
);
#24820=SHAPE_DEFINITION_REPRESENTATION(#24832,#24860);
#24832=PRODUCT_DEFINITION_SHAPE('',$,#24873);
#24860=SHAPE_REPRESENTATION('',(#10261),#24803);
#24866=PRODUCT_DEFINITION_CONTEXT('part definition',#24904,'design');
#24873=PRODUCT_DEFINITION('2026-11-10-05-11-11-294',
'Upper structural shell',#24885,#24866);
#24885=PRODUCT_DEFINITION_FORMATION('',$,#24912);
#24904=APPLICATION_CONTEXT(
'Core Data for Automotive Mechanical Design Process');
#24905=PRODUCT_CONTEXT('part definition',#24904,'mechanical');
#24912=PRODUCT('2026-11-10-05-11-11-294','Upper structural shell',$,(#24905));
#24922=PRESENTATION_STYLE_ASSIGNMENT((#24930));
#24930=SURFACE_STYLE_USAGE(.BOTH.,#24938);
#24938=SURFACE_SIDE_STYLE('',(#24946));
#24946=SURFACE_STYLE_FILL_AREA(#24954);
#24954=FILL_AREA_STYLE('Structural dark blue',(#24962));
#24962=FILL_AREA_STYLE_COLOUR('Structural dark blue',#24970);
#24970=COLOUR_RGB('Structural dark blue',0.0901960784313725,0.270588235294118,
0.513725490196078);
ENDSEC;
END-ISO-10303-21;
